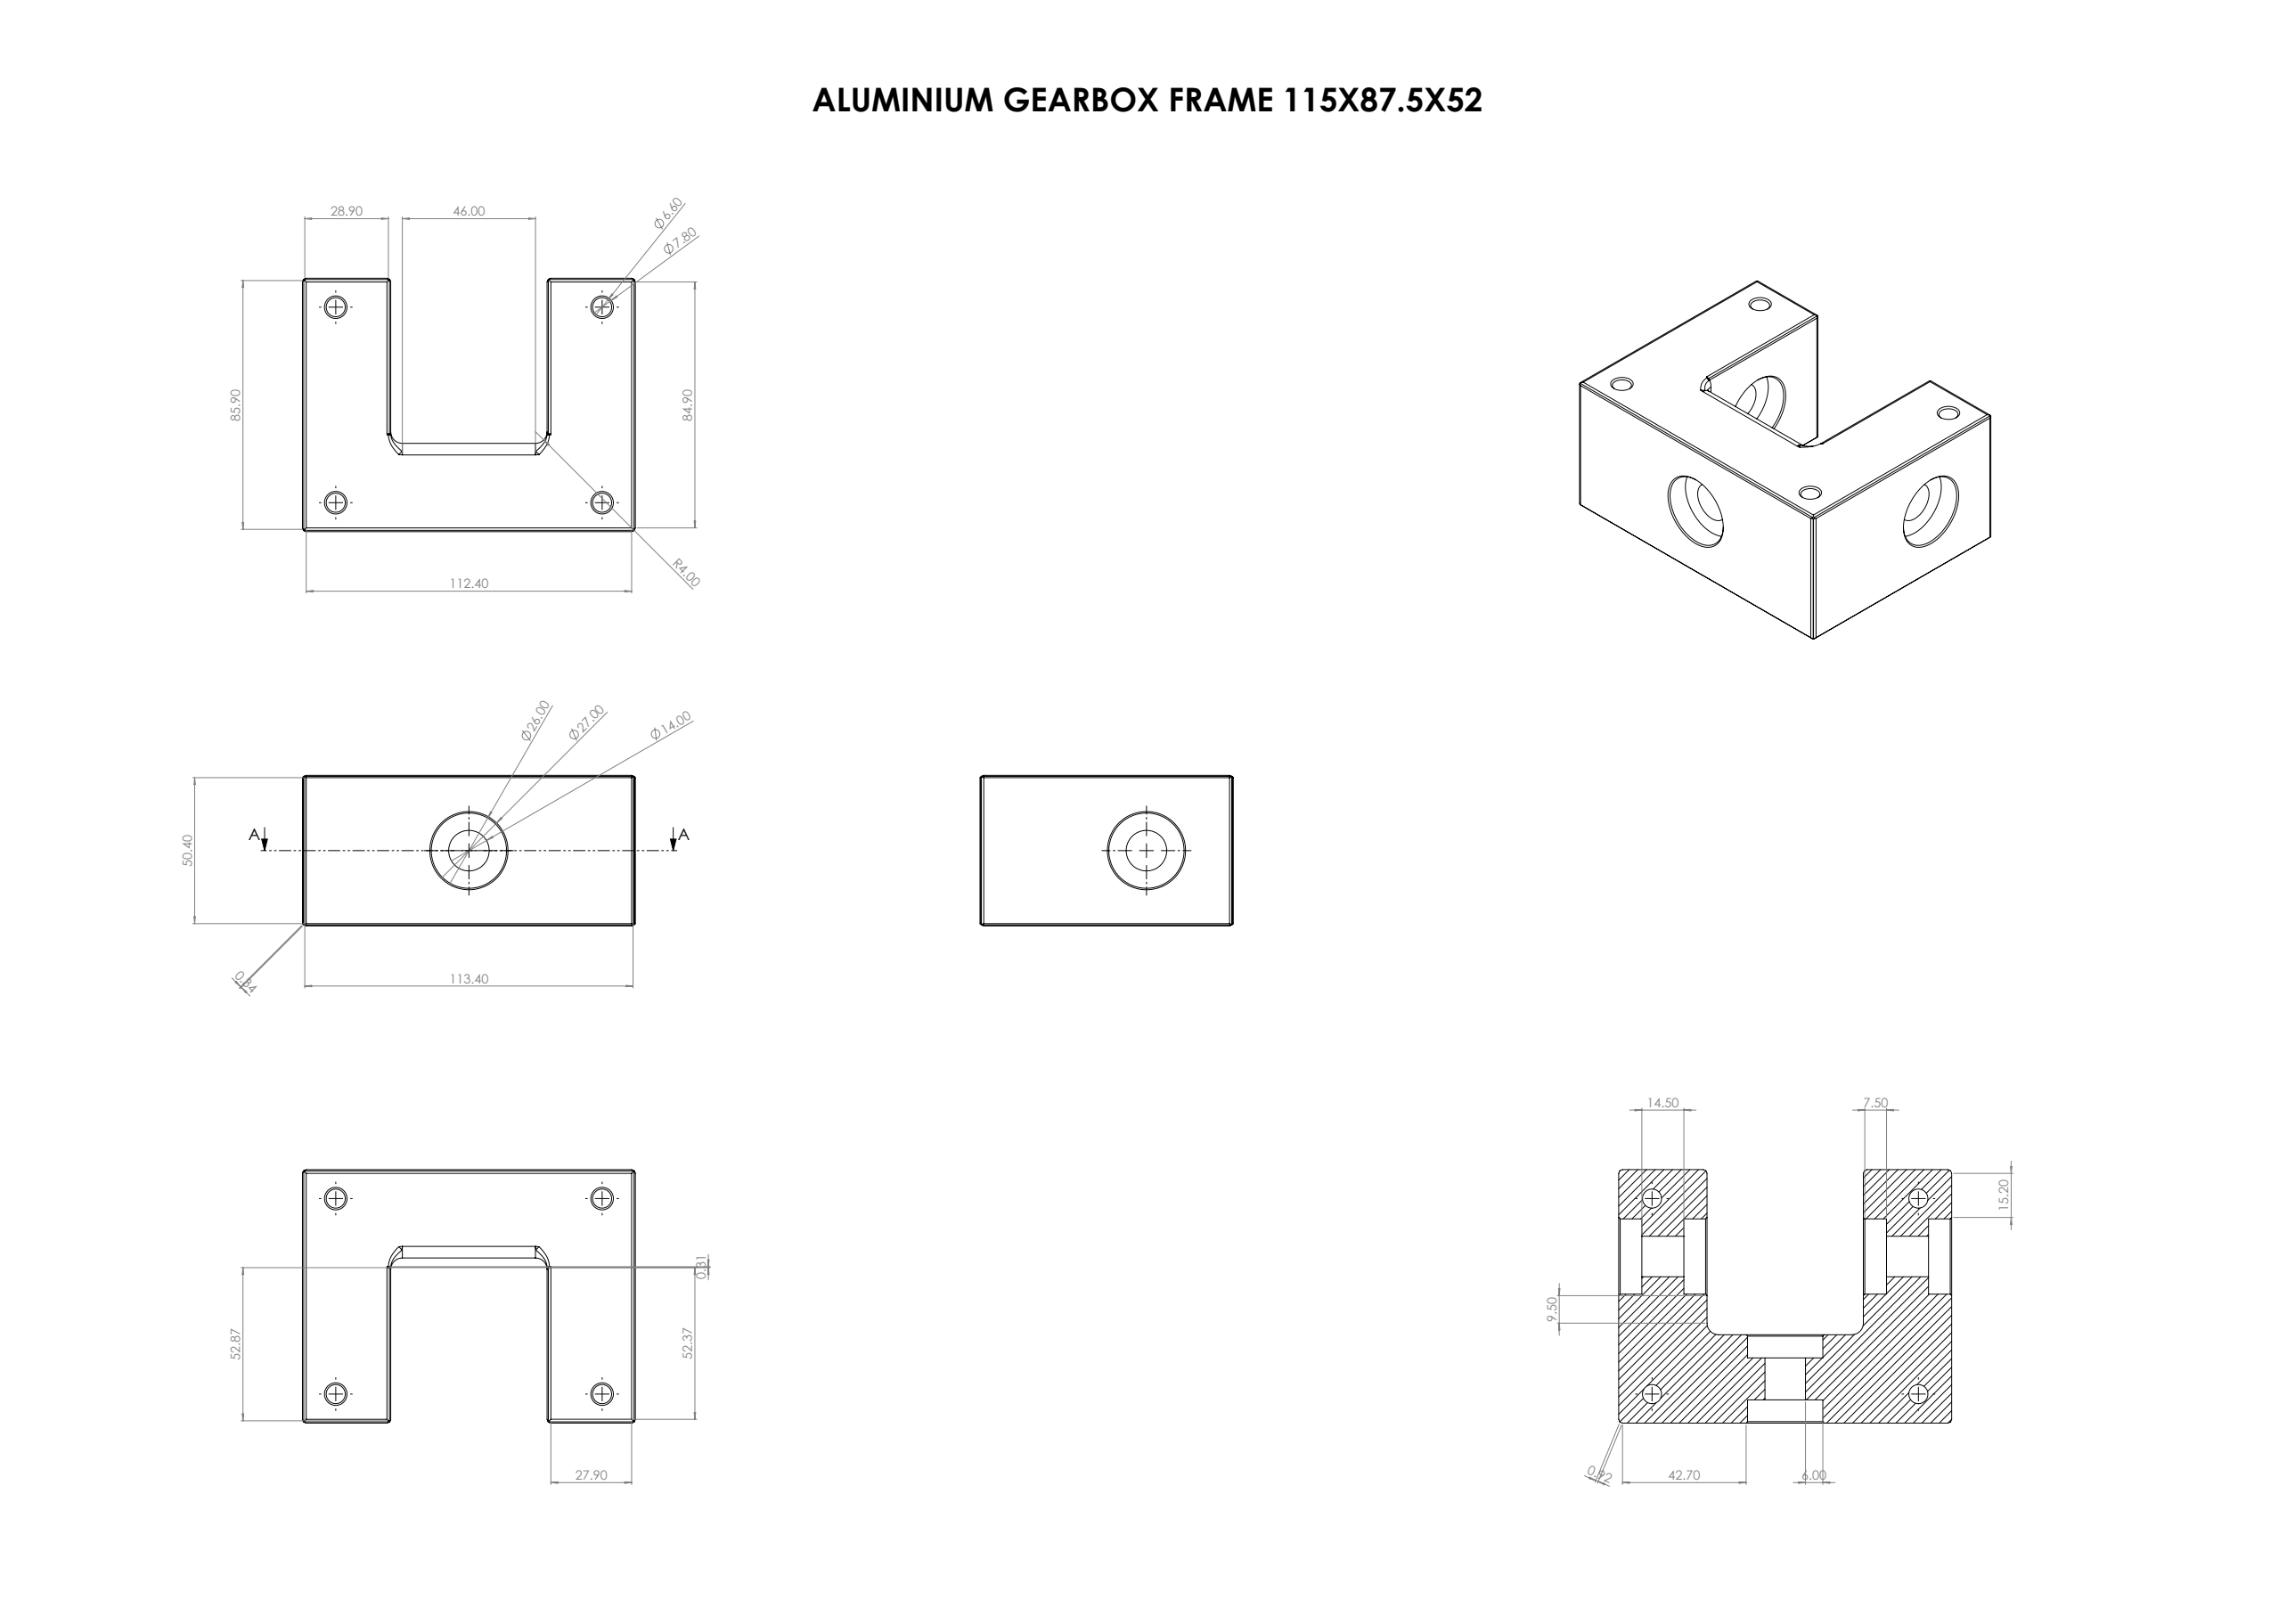
ISO-10303-21;
HEADER;
/* Generated by software containing ST-Developer
 * from STEP Tools, Inc. (www.steptools.com) 
 */

FILE_DESCRIPTION(
/* description */ (''),
/* implementation_level */ '2;1');

FILE_NAME(
/* name */ 
'01_Aluminium_Gearbox_Frame_115x87.5x52.step',
/* time_stamp */ '2026-10-22T00:21:42-07:00',
/* author */ (''),
/* organization */ (''),
/* preprocessor_version */ 'ST-DEVELOPER v20.2',
/* originating_system */ 'Autodesk Translation Framework v15.15.0.0',
/* authorisation */ '');

FILE_SCHEMA (('AUTOMOTIVE_DESIGN { 1 0 10303 214 3 1 1 }'));
ENDSEC;

DATA;
#10=MECHANICAL_DESIGN_GEOMETRIC_PRESENTATION_REPRESENTATION('',(#205),#31638);
#183=SHAPE_REPRESENTATION_RELATIONSHIP('SRR','None',#31705,#194);
#194=ADVANCED_BREP_SHAPE_REPRESENTATION('',(#216),#31627);
#205=STYLED_ITEM('',(#31809),#216);
#216=MANIFOLD_SOLID_BREP('Frame',#12480);
#227=TOROIDAL_SURFACE('',#12758,0.8,0.4);
#228=TOROIDAL_SURFACE('',#12761,0.8,0.4);
#229=TOROIDAL_SURFACE('',#12765,0.8,0.4);
#230=TOROIDAL_SURFACE('',#12770,0.8,0.4);
#246=CYLINDRICAL_SURFACE('',#12692,0.33);
#247=CYLINDRICAL_SURFACE('',#12697,0.33);
#248=CYLINDRICAL_SURFACE('',#12702,0.33);
#249=CYLINDRICAL_SURFACE('',#12707,0.33);
#250=CYLINDRICAL_SURFACE('',#12713,1.3);
#251=CYLINDRICAL_SURFACE('',#12717,0.7);
#252=CYLINDRICAL_SURFACE('',#12721,1.3);
#253=CYLINDRICAL_SURFACE('',#12727,1.3);
#254=CYLINDRICAL_SURFACE('',#12731,0.7);
#255=CYLINDRICAL_SURFACE('',#12735,1.3);
#256=CYLINDRICAL_SURFACE('',#12740,1.3);
#257=CYLINDRICAL_SURFACE('',#12744,0.7);
#258=CYLINDRICAL_SURFACE('',#12748,1.3);
#259=CYLINDRICAL_SURFACE('',#12768,0.4);
#260=CYLINDRICAL_SURFACE('',#12772,0.4);
#261=CYLINDRICAL_SURFACE('',#12773,0.4);
#262=CYLINDRICAL_SURFACE('',#12775,0.4);
#362=CONICAL_SURFACE('',#12690,0.36,0.785398163397444);
#363=CONICAL_SURFACE('',#12694,0.36,0.785398163397444);
#364=CONICAL_SURFACE('',#12695,0.36,0.785398163397444);
#365=CONICAL_SURFACE('',#12699,0.36,0.785398163397444);
#366=CONICAL_SURFACE('',#12700,0.36,0.785398163397444);
#367=CONICAL_SURFACE('',#12704,0.36,0.785398163397444);
#368=CONICAL_SURFACE('',#12705,0.36,0.785398163397444);
#369=CONICAL_SURFACE('',#12709,0.36,0.785398163397444);
#370=CONICAL_SURFACE('',#12710,1.35,0.78539816339745);
#371=CONICAL_SURFACE('',#12723,1.35,0.785398163397441);
#372=CONICAL_SURFACE('',#12725,1.35,0.785398163397451);
#373=CONICAL_SURFACE('',#12737,1.35,0.785398163397453);
#374=CONICAL_SURFACE('',#12738,1.35,0.785398163397453);
#375=CONICAL_SURFACE('',#12750,1.35,0.785398163397451);
#457=B_SPLINE_CURVE_WITH_KNOTS('',3,(#16701,#16702,#16703,#16704),
 .UNSPECIFIED.,.F.,.F.,(4,4),(0.,1.),.UNSPECIFIED.);
#458=B_SPLINE_CURVE_WITH_KNOTS('',3,(#16705,#16706,#16707,#16708),
 .UNSPECIFIED.,.F.,.F.,(4,4),(-5.39792313687514,-5.36678788880707),
 .UNSPECIFIED.);
#459=B_SPLINE_CURVE_WITH_KNOTS('',3,(#16709,#16710,#16711,#16712),
 .UNSPECIFIED.,.F.,.F.,(4,4),(5.36678788880707,5.39792313687514),
 .UNSPECIFIED.);
#460=B_SPLINE_CURVE_WITH_KNOTS('',3,(#16730,#16731,#16732,#16733),
 .UNSPECIFIED.,.F.,.F.,(4,4),(0.,1.),.UNSPECIFIED.);
#461=B_SPLINE_CURVE_WITH_KNOTS('',3,(#16734,#16735,#16736,#16737),
 .UNSPECIFIED.,.F.,.F.,(4,4),(-1.,0.),.UNSPECIFIED.);
#462=B_SPLINE_CURVE_WITH_KNOTS('',3,(#16740,#16741,#16742,#16743,#16744,
#16745,#16746,#16747,#16748),.UNSPECIFIED.,.F.,.F.,(4,1,1,1,1,1,4),(0.0919588831913347,
0.287428968788757,0.385164011587469,0.48289905438618,0.580634097184891,
0.678369139983603,0.776104182782314),.UNSPECIFIED.);
#463=B_SPLINE_CURVE_WITH_KNOTS('',3,(#16750,#16751,#16752,#16753),
 .UNSPECIFIED.,.F.,.F.,(4,4),(-1.,0.),.UNSPECIFIED.);
#464=B_SPLINE_CURVE_WITH_KNOTS('',3,(#16757,#16758,#16759,#16760),
 .UNSPECIFIED.,.F.,.F.,(4,4),(0.,1.),.UNSPECIFIED.);
#465=B_SPLINE_CURVE_WITH_KNOTS('',3,(#16762,#16763,#16764,#16765,#16766,
#16767,#16768,#16769,#16770),.UNSPECIFIED.,.F.,.F.,(4,1,1,1,2,4),(2.02212896015404,
2.13032466905734,2.23852037796064,2.34671608686394,2.56310750467053,2.7062742594363),
 .UNSPECIFIED.);
#466=B_SPLINE_CURVE_WITH_KNOTS('',3,(#16772,#16773,#16774,#16775),
 .UNSPECIFIED.,.F.,.F.,(4,4),(0.,1.),.UNSPECIFIED.);
#467=B_SPLINE_CURVE_WITH_KNOTS('',3,(#16777,#16778,#16779,#16780),
 .UNSPECIFIED.,.F.,.F.,(4,4),(-0.333212111192934,-0.302076863348255),
 .UNSPECIFIED.);
#468=B_SPLINE_CURVE_WITH_KNOTS('',3,(#16816,#16817,#16818,#16819),
 .UNSPECIFIED.,.F.,.F.,(4,4),(5.36678788880707,5.40717967697245),
 .UNSPECIFIED.);
#469=B_SPLINE_CURVE_WITH_KNOTS('',3,(#16848,#16849,#16850,#16851),
 .UNSPECIFIED.,.F.,.F.,(4,4),(-1.,0.),.UNSPECIFIED.);
#470=B_SPLINE_CURVE_WITH_KNOTS('',3,(#16852,#16853,#16854,#16855),
 .UNSPECIFIED.,.F.,.F.,(4,4),(0.302076863348255,0.333212111192934),
 .UNSPECIFIED.);
#471=B_SPLINE_CURVE_WITH_KNOTS('',3,(#16872,#16873,#16874,#16875),
 .UNSPECIFIED.,.F.,.F.,(4,4),(-1.,0.),.UNSPECIFIED.);
#472=B_SPLINE_CURVE_WITH_KNOTS('',3,(#16906,#16907,#16908,#16909),
 .UNSPECIFIED.,.F.,.F.,(4,4),(0.,1.),.UNSPECIFIED.);
#473=B_SPLINE_CURVE_WITH_KNOTS('',3,(#16910,#16911,#16912,#16913),
 .UNSPECIFIED.,.F.,.F.,(4,4),(0.302076863124856,0.333212111192934),
 .UNSPECIFIED.);
#474=B_SPLINE_CURVE_WITH_KNOTS('',3,(#16914,#16915,#16916,#16917),
 .UNSPECIFIED.,.F.,.F.,(4,4),(-0.333212111192934,-0.302076863124856),
 .UNSPECIFIED.);
#475=B_SPLINE_CURVE_WITH_KNOTS('',3,(#16935,#16936,#16937,#16938),
 .UNSPECIFIED.,.F.,.F.,(4,4),(0.,1.),.UNSPECIFIED.);
#476=B_SPLINE_CURVE_WITH_KNOTS('',3,(#16939,#16940,#16941,#16942),
 .UNSPECIFIED.,.F.,.F.,(4,4),(-1.,0.),.UNSPECIFIED.);
#477=B_SPLINE_CURVE_WITH_KNOTS('',3,(#16945,#16946,#16947,#16948,#16949,
#16950,#16951,#16952),.UNSPECIFIED.,.F.,.F.,(4,1,1,1,1,4),(0.091958883192206,
0.287428968789379,0.482899054386553,0.531766575785846,0.678369139983726,
0.776104182782313),.UNSPECIFIED.);
#478=B_SPLINE_CURVE_WITH_KNOTS('',3,(#16954,#16955,#16956,#16957),
 .UNSPECIFIED.,.F.,.F.,(4,4),(-1.,0.),.UNSPECIFIED.);
#479=B_SPLINE_CURVE_WITH_KNOTS('',3,(#16961,#16962,#16963,#16964),
 .UNSPECIFIED.,.F.,.F.,(4,4),(0.,1.),.UNSPECIFIED.);
#480=B_SPLINE_CURVE_WITH_KNOTS('',3,(#16966,#16967,#16968,#16969,#16970,
#16971,#16972,#16973,#16974),.UNSPECIFIED.,.F.,.F.,(4,1,1,1,2,4),(2.02212896015404,
2.13032466905734,2.23852037796064,2.34671608686394,2.56310750467053,2.70627425943714),
 .UNSPECIFIED.);
#481=B_SPLINE_CURVE_WITH_KNOTS('',3,(#16976,#16977,#16978,#16979),
 .UNSPECIFIED.,.F.,.F.,(4,4),(0.,1.),.UNSPECIFIED.);
#482=B_SPLINE_CURVE_WITH_KNOTS('',3,(#16981,#16982,#16983,#16984),
 .UNSPECIFIED.,.F.,.F.,(4,4),(5.36678788880707,5.39792313665175),
 .UNSPECIFIED.);
#483=B_SPLINE_CURVE_WITH_KNOTS('',3,(#17020,#17021,#17022,#17023),
 .UNSPECIFIED.,.F.,.F.,(4,4),(-0.333212111192934,-0.292820323027551),
 .UNSPECIFIED.);
#484=B_SPLINE_CURVE_WITH_KNOTS('',3,(#17057,#17058,#17059,#17060),
 .UNSPECIFIED.,.F.,.F.,(4,4),(-1.,0.),.UNSPECIFIED.);
#485=B_SPLINE_CURVE_WITH_KNOTS('',3,(#17061,#17062,#17063,#17064),
 .UNSPECIFIED.,.F.,.F.,(4,4),(-5.39792313665175,-5.36678788880707),
 .UNSPECIFIED.);
#486=B_SPLINE_CURVE_WITH_KNOTS('',3,(#17081,#17082,#17083,#17084),
 .UNSPECIFIED.,.F.,.F.,(4,4),(-1.,0.),.UNSPECIFIED.);
#487=B_SPLINE_CURVE_WITH_KNOTS('',3,(#17238,#17239,#17240,#17241),
 .UNSPECIFIED.,.F.,.F.,(4,4),(0.,1.),.UNSPECIFIED.);
#488=B_SPLINE_CURVE_WITH_KNOTS('',3,(#17242,#17243,#17244,#17245,#17246,
#17247,#17248,#17249,#17250),.UNSPECIFIED.,.F.,.F.,(4,1,1,1,1,1,4),(-0.776104182782314,
-0.678369139983603,-0.580634097184891,-0.48289905438618,-0.385164011587469,
-0.287428968788757,-0.0919588831913347),.UNSPECIFIED.);
#489=B_SPLINE_CURVE_WITH_KNOTS('',3,(#17284,#17285,#17286,#17287),
 .UNSPECIFIED.,.F.,.F.,(4,4),(0.,1.),.UNSPECIFIED.);
#490=B_SPLINE_CURVE_WITH_KNOTS('',3,(#17288,#17289,#17290,#17291,#17292,
#17293,#17294,#17295),.UNSPECIFIED.,.F.,.F.,(4,1,1,1,1,4),(-0.776104182782313,
-0.678369139983726,-0.531766575785846,-0.482899054386553,-0.287428968789379,
-0.091958883192206),.UNSPECIFIED.);
#491=B_SPLINE_CURVE_WITH_KNOTS('',3,(#17340,#17341,#17342,#17343),
 .UNSPECIFIED.,.F.,.F.,(4,4),(-1.,0.),.UNSPECIFIED.);
#492=B_SPLINE_CURVE_WITH_KNOTS('',3,(#17345,#17346,#17347,#17348,#17349,
#17350,#17351,#17352,#17353),.UNSPECIFIED.,.F.,.F.,(4,2,1,1,1,4),(-2.7062742594363,
-2.56310750467053,-2.34671608686394,-2.23852037796064,-2.13032466905734,
-2.02212896015404),.UNSPECIFIED.);
#493=B_SPLINE_CURVE_WITH_KNOTS('',3,(#17371,#17372,#17373,#17374),
 .UNSPECIFIED.,.F.,.F.,(4,4),(0.292820323027551,0.333212111192934),
 .UNSPECIFIED.);
#494=B_SPLINE_CURVE_WITH_KNOTS('',3,(#17412,#17413,#17414,#17415),
 .UNSPECIFIED.,.F.,.F.,(4,4),(-1.,0.),.UNSPECIFIED.);
#495=B_SPLINE_CURVE_WITH_KNOTS('',3,(#17417,#17418,#17419,#17420,#17421,
#17422,#17423,#17424,#17425),.UNSPECIFIED.,.F.,.F.,(4,2,1,1,1,4),(-2.70627425943714,
-2.56310750467053,-2.34671608686394,-2.23852037796064,-2.13032466905734,
-2.02212896015404),.UNSPECIFIED.);
#496=B_SPLINE_CURVE_WITH_KNOTS('',3,(#17443,#17444,#17445,#17446),
 .UNSPECIFIED.,.F.,.F.,(4,4),(-5.40717967697245,-5.36678788880707),
 .UNSPECIFIED.);
#497=B_SPLINE_CURVE_WITH_KNOTS('',3,(#17463,#17464,#17465,#17466),
 .UNSPECIFIED.,.F.,.F.,(4,4),(0.,1.),.UNSPECIFIED.);
#498=B_SPLINE_CURVE_WITH_KNOTS('',3,(#17483,#17484,#17485,#17486),
 .UNSPECIFIED.,.F.,.F.,(4,4),(0.,1.),.UNSPECIFIED.);
#499=B_SPLINE_CURVE_WITH_KNOTS('',3,(#17503,#17504,#17505,#17506),
 .UNSPECIFIED.,.F.,.F.,(4,4),(-1.,0.),.UNSPECIFIED.);
#500=B_SPLINE_CURVE_WITH_KNOTS('',3,(#17523,#17524,#17525,#17526),
 .UNSPECIFIED.,.F.,.F.,(4,4),(-1.,0.),.UNSPECIFIED.);
#1186=B_SPLINE_SURFACE_WITH_KNOTS('',3,3,((#16683,#16684,#16685,#16686),
(#16687,#16688,#16689,#16690),(#16691,#16692,#16693,#16694),(#16695,#16696,
#16697,#16698)),.UNSPECIFIED.,.F.,.F.,.F.,(4,4),(4,4),(0.,1.),(-5.39792313687514,
-5.36678788880707),.UNSPECIFIED.);
#1187=B_SPLINE_SURFACE_WITH_KNOTS('',3,3,((#16713,#16714,#16715,#16716),
(#16717,#16718,#16719,#16720),(#16721,#16722,#16723,#16724),(#16725,#16726,
#16727,#16728)),.UNSPECIFIED.,.F.,.F.,.F.,(4,4),(4,4),(0.,1.),(0.,1.),
 .UNSPECIFIED.);
#1188=B_SPLINE_SURFACE_WITH_KNOTS('',3,3,((#16798,#16799,#16800,#16801),
(#16802,#16803,#16804,#16805),(#16806,#16807,#16808,#16809),(#16810,#16811,
#16812,#16813)),.UNSPECIFIED.,.F.,.F.,.F.,(4,4),(4,4),(0.,1.),(-5.40717967697245,
-5.36678788880707),.UNSPECIFIED.);
#1189=B_SPLINE_SURFACE_WITH_KNOTS('',3,3,((#16831,#16832,#16833,#16834),
(#16835,#16836,#16837,#16838),(#16839,#16840,#16841,#16842),(#16843,#16844,
#16845,#16846)),.UNSPECIFIED.,.F.,.F.,.F.,(4,4),(4,4),(0.,1.),(-0.333212111192934,
-0.302076863348255),.UNSPECIFIED.);
#1190=B_SPLINE_SURFACE_WITH_KNOTS('',3,3,((#16856,#16857,#16858,#16859),
(#16860,#16861,#16862,#16863),(#16864,#16865,#16866,#16867),(#16868,#16869,
#16870,#16871)),.UNSPECIFIED.,.F.,.F.,.F.,(4,4),(4,4),(0.,1.),(0.,1.),
 .UNSPECIFIED.);
#1191=B_SPLINE_SURFACE_WITH_KNOTS('',3,3,((#16888,#16889,#16890,#16891),
(#16892,#16893,#16894,#16895),(#16896,#16897,#16898,#16899),(#16900,#16901,
#16902,#16903)),.UNSPECIFIED.,.F.,.F.,.F.,(4,4),(4,4),(0.,1.),(0.302076863124856,
0.333212111192934),.UNSPECIFIED.);
#1192=B_SPLINE_SURFACE_WITH_KNOTS('',3,3,((#16918,#16919,#16920,#16921),
(#16922,#16923,#16924,#16925),(#16926,#16927,#16928,#16929),(#16930,#16931,
#16932,#16933)),.UNSPECIFIED.,.F.,.F.,.F.,(4,4),(4,4),(0.,1.),(0.,1.),
 .UNSPECIFIED.);
#1193=B_SPLINE_SURFACE_WITH_KNOTS('',3,3,((#17002,#17003,#17004,#17005),
(#17006,#17007,#17008,#17009),(#17010,#17011,#17012,#17013),(#17014,#17015,
#17016,#17017)),.UNSPECIFIED.,.F.,.F.,.F.,(4,4),(4,4),(0.,1.),(0.292820323027551,
0.333212111192934),.UNSPECIFIED.);
#1194=B_SPLINE_SURFACE_WITH_KNOTS('',3,3,((#17040,#17041,#17042,#17043),
(#17044,#17045,#17046,#17047),(#17048,#17049,#17050,#17051),(#17052,#17053,
#17054,#17055)),.UNSPECIFIED.,.F.,.F.,.F.,(4,4),(4,4),(0.,1.),(5.36678788880707,
5.39792313665175),.UNSPECIFIED.);
#1195=B_SPLINE_SURFACE_WITH_KNOTS('',3,3,((#17065,#17066,#17067,#17068),
(#17069,#17070,#17071,#17072),(#17073,#17074,#17075,#17076),(#17077,#17078,
#17079,#17080)),.UNSPECIFIED.,.F.,.F.,.F.,(4,4),(4,4),(0.,1.),(0.,1.),
 .UNSPECIFIED.);
#1196=B_SPLINE_SURFACE_WITH_KNOTS('',3,3,((#17201,#17202,#17203,#17204,
#17205,#17206,#17207,#17208,#17209),(#17210,#17211,#17212,#17213,#17214,
#17215,#17216,#17217,#17218),(#17219,#17220,#17221,#17222,#17223,#17224,
#17225,#17226,#17227),(#17228,#17229,#17230,#17231,#17232,#17233,#17234,
#17235,#17236)),.UNSPECIFIED.,.F.,.F.,.F.,(4,4),(4,1,1,1,1,1,4),(0.,1.),
(0.0919588831913347,0.287428968788757,0.385164011587469,0.48289905438618,
0.580634097184891,0.678369139983603,0.776104182782314),.UNSPECIFIED.);
#1197=B_SPLINE_SURFACE_WITH_KNOTS('',3,3,((#17251,#17252,#17253,#17254,
#17255,#17256,#17257,#17258),(#17259,#17260,#17261,#17262,#17263,#17264,
#17265,#17266),(#17267,#17268,#17269,#17270,#17271,#17272,#17273,#17274),
(#17275,#17276,#17277,#17278,#17279,#17280,#17281,#17282)),
 .UNSPECIFIED.,.F.,.F.,.F.,(4,4),(4,1,1,1,1,4),(0.,1.),(0.091958883192206,
0.287428968789379,0.482899054386553,0.531766575785846,0.678369139983726,
0.776104182782313),.UNSPECIFIED.);
#1198=B_SPLINE_SURFACE_WITH_KNOTS('',3,3,((#17303,#17304,#17305,#17306,
#17307,#17308,#17309,#17310,#17311),(#17312,#17313,#17314,#17315,#17316,
#17317,#17318,#17319,#17320),(#17321,#17322,#17323,#17324,#17325,#17326,
#17327,#17328,#17329),(#17330,#17331,#17332,#17333,#17334,#17335,#17336,
#17337,#17338)),.UNSPECIFIED.,.F.,.F.,.F.,(4,4),(4,1,1,1,2,4),(0.,1.),(2.02212896015404,
2.13032466905734,2.23852037796064,2.34671608686394,2.56310750467053,2.7062742594363),
 .UNSPECIFIED.);
#1199=B_SPLINE_SURFACE_WITH_KNOTS('',3,3,((#17355,#17356,#17357,#17358),
(#17359,#17360,#17361,#17362),(#17363,#17364,#17365,#17366),(#17367,#17368,
#17369,#17370)),.UNSPECIFIED.,.F.,.F.,.F.,(4,4),(4,4),(0.,1.),(-0.333212111192934,
-0.292820323027551),.UNSPECIFIED.);
#1200=B_SPLINE_SURFACE_WITH_KNOTS('',3,3,((#17375,#17376,#17377,#17378,
#17379,#17380,#17381,#17382,#17383),(#17384,#17385,#17386,#17387,#17388,
#17389,#17390,#17391,#17392),(#17393,#17394,#17395,#17396,#17397,#17398,
#17399,#17400,#17401),(#17402,#17403,#17404,#17405,#17406,#17407,#17408,
#17409,#17410)),.UNSPECIFIED.,.F.,.F.,.F.,(4,4),(4,1,1,1,2,4),(0.,1.),(2.02212896015404,
2.13032466905734,2.23852037796064,2.34671608686394,2.56310750467053,2.70627425943714),
 .UNSPECIFIED.);
#1201=B_SPLINE_SURFACE_WITH_KNOTS('',3,3,((#17427,#17428,#17429,#17430),
(#17431,#17432,#17433,#17434),(#17435,#17436,#17437,#17438),(#17439,#17440,
#17441,#17442)),.UNSPECIFIED.,.F.,.F.,.F.,(4,4),(4,4),(0.,1.),(5.36678788880707,
5.40717967697245),.UNSPECIFIED.);
#1202=B_SPLINE_SURFACE_WITH_KNOTS('',3,3,((#17447,#17448,#17449,#17450),
(#17451,#17452,#17453,#17454),(#17455,#17456,#17457,#17458),(#17459,#17460,
#17461,#17462)),.UNSPECIFIED.,.F.,.F.,.F.,(4,4),(4,4),(0.,1.),(0.,1.),
 .UNSPECIFIED.);
#1203=B_SPLINE_SURFACE_WITH_KNOTS('',3,3,((#17467,#17468,#17469,#17470),
(#17471,#17472,#17473,#17474),(#17475,#17476,#17477,#17478),(#17479,#17480,
#17481,#17482)),.UNSPECIFIED.,.F.,.F.,.F.,(4,4),(4,4),(0.,1.),(0.,1.),
 .UNSPECIFIED.);
#1204=B_SPLINE_SURFACE_WITH_KNOTS('',3,3,((#17487,#17488,#17489,#17490),
(#17491,#17492,#17493,#17494),(#17495,#17496,#17497,#17498),(#17499,#17500,
#17501,#17502)),.UNSPECIFIED.,.F.,.F.,.F.,(4,4),(4,4),(0.,1.),(0.,1.),
 .UNSPECIFIED.);
#1205=B_SPLINE_SURFACE_WITH_KNOTS('',3,3,((#17507,#17508,#17509,#17510),
(#17511,#17512,#17513,#17514),(#17515,#17516,#17517,#17518),(#17519,#17520,
#17521,#17522)),.UNSPECIFIED.,.F.,.F.,.F.,(4,4),(4,4),(0.,1.),(0.,1.),
 .UNSPECIFIED.);
#1340=FACE_BOUND('',#2515,.T.);
#1341=FACE_BOUND('',#2527,.T.);
#1342=FACE_BOUND('',#2540,.T.);
#1343=FACE_BOUND('',#2556,.T.);
#1344=FACE_BOUND('',#2564,.T.);
#1345=FACE_BOUND('',#2565,.T.);
#1346=FACE_BOUND('',#2566,.T.);
#1347=FACE_BOUND('',#2567,.T.);
#1348=FACE_BOUND('',#2581,.T.);
#1349=FACE_BOUND('',#2582,.T.);
#1350=FACE_BOUND('',#2583,.T.);
#1351=FACE_BOUND('',#2584,.T.);
#1352=FACE_BOUND('',#2609,.T.);
#1353=FACE_BOUND('',#2612,.T.);
#1354=FACE_BOUND('',#2618,.T.);
#1355=FACE_BOUND('',#2621,.T.);
#1356=FACE_BOUND('',#2627,.T.);
#1357=FACE_BOUND('',#2630,.T.);
#1358=FACE_BOUND('',#2653,.T.);
#1359=FACE_BOUND('',#2660,.T.);
#1405=CIRCLE('',#12617,0.8);
#1406=CIRCLE('',#12618,0.8);
#1407=CIRCLE('',#12619,1.35);
#1408=CIRCLE('',#12631,1.35);
#1409=CIRCLE('',#12644,1.35);
#1410=CIRCLE('',#12660,0.8);
#1411=CIRCLE('',#12661,0.8);
#1412=CIRCLE('',#12662,1.35);
#1413=CIRCLE('',#12668,0.39);
#1414=CIRCLE('',#12669,0.39);
#1415=CIRCLE('',#12670,0.39);
#1416=CIRCLE('',#12671,0.39);
#1417=CIRCLE('',#12680,0.39);
#1418=CIRCLE('',#12681,0.39);
#1419=CIRCLE('',#12682,0.39);
#1420=CIRCLE('',#12683,0.39);
#1421=CIRCLE('',#12691,0.33);
#1422=CIRCLE('',#12693,0.33);
#1423=CIRCLE('',#12696,0.33);
#1424=CIRCLE('',#12698,0.33);
#1425=CIRCLE('',#12701,0.33);
#1426=CIRCLE('',#12703,0.33);
#1427=CIRCLE('',#12706,0.33);
#1428=CIRCLE('',#12708,0.33);
#1429=CIRCLE('',#12711,1.35);
#1430=CIRCLE('',#12712,1.3);
#1431=CIRCLE('',#12714,1.3);
#1432=CIRCLE('',#12716,0.7);
#1433=CIRCLE('',#12718,0.7);
#1434=CIRCLE('',#12720,1.3);
#1435=CIRCLE('',#12722,1.3);
#1436=CIRCLE('',#12724,1.35);
#1437=CIRCLE('',#12726,1.3);
#1438=CIRCLE('',#12728,1.3);
#1439=CIRCLE('',#12730,0.7);
#1440=CIRCLE('',#12732,0.7);
#1441=CIRCLE('',#12734,1.3);
#1442=CIRCLE('',#12736,1.3);
#1443=CIRCLE('',#12739,1.3);
#1444=CIRCLE('',#12741,1.3);
#1445=CIRCLE('',#12743,0.7);
#1446=CIRCLE('',#12745,0.7);
#1447=CIRCLE('',#12747,1.3);
#1448=CIRCLE('',#12749,1.3);
#1449=CIRCLE('',#12759,0.4);
#1450=CIRCLE('',#12760,0.4);
#1451=CIRCLE('',#12762,0.4);
#1452=CIRCLE('',#12763,0.4);
#1453=CIRCLE('',#12766,0.4);
#1454=CIRCLE('',#12767,0.4);
#1455=CIRCLE('',#12769,0.4);
#1456=CIRCLE('',#12771,0.4);
#1819=FACE_OUTER_BOUND('',#2513,.T.);
#1820=FACE_OUTER_BOUND('',#2514,.T.);
#1821=FACE_OUTER_BOUND('',#2516,.T.);
#1822=FACE_OUTER_BOUND('',#2517,.T.);
#1823=FACE_OUTER_BOUND('',#2518,.T.);
#1824=FACE_OUTER_BOUND('',#2519,.T.);
#1825=FACE_OUTER_BOUND('',#2520,.T.);
#1826=FACE_OUTER_BOUND('',#2521,.T.);
#1827=FACE_OUTER_BOUND('',#2522,.T.);
#1828=FACE_OUTER_BOUND('',#2523,.T.);
#1829=FACE_OUTER_BOUND('',#2524,.T.);
#1830=FACE_OUTER_BOUND('',#2525,.T.);
#1831=FACE_OUTER_BOUND('',#2526,.T.);
#1832=FACE_OUTER_BOUND('',#2528,.T.);
#1833=FACE_OUTER_BOUND('',#2529,.T.);
#1834=FACE_OUTER_BOUND('',#2530,.T.);
#1835=FACE_OUTER_BOUND('',#2531,.T.);
#1836=FACE_OUTER_BOUND('',#2532,.T.);
#1837=FACE_OUTER_BOUND('',#2533,.T.);
#1838=FACE_OUTER_BOUND('',#2534,.T.);
#1839=FACE_OUTER_BOUND('',#2535,.T.);
#1840=FACE_OUTER_BOUND('',#2536,.T.);
#1841=FACE_OUTER_BOUND('',#2537,.T.);
#1842=FACE_OUTER_BOUND('',#2538,.T.);
#1843=FACE_OUTER_BOUND('',#2539,.T.);
#1844=FACE_OUTER_BOUND('',#2541,.T.);
#1845=FACE_OUTER_BOUND('',#2542,.T.);
#1846=FACE_OUTER_BOUND('',#2543,.T.);
#1847=FACE_OUTER_BOUND('',#2544,.T.);
#1848=FACE_OUTER_BOUND('',#2545,.T.);
#1849=FACE_OUTER_BOUND('',#2546,.T.);
#1850=FACE_OUTER_BOUND('',#2547,.T.);
#1851=FACE_OUTER_BOUND('',#2548,.T.);
#1852=FACE_OUTER_BOUND('',#2549,.T.);
#1853=FACE_OUTER_BOUND('',#2550,.T.);
#1854=FACE_OUTER_BOUND('',#2551,.T.);
#1855=FACE_OUTER_BOUND('',#2552,.T.);
#1856=FACE_OUTER_BOUND('',#2553,.T.);
#1857=FACE_OUTER_BOUND('',#2554,.T.);
#1858=FACE_OUTER_BOUND('',#2555,.T.);
#1859=FACE_OUTER_BOUND('',#2557,.T.);
#1860=FACE_OUTER_BOUND('',#2558,.T.);
#1861=FACE_OUTER_BOUND('',#2559,.T.);
#1862=FACE_OUTER_BOUND('',#2560,.T.);
#1863=FACE_OUTER_BOUND('',#2561,.T.);
#1864=FACE_OUTER_BOUND('',#2562,.T.);
#1865=FACE_OUTER_BOUND('',#2563,.T.);
#1866=FACE_OUTER_BOUND('',#2568,.T.);
#1867=FACE_OUTER_BOUND('',#2569,.T.);
#1868=FACE_OUTER_BOUND('',#2570,.T.);
#1869=FACE_OUTER_BOUND('',#2571,.T.);
#1870=FACE_OUTER_BOUND('',#2572,.T.);
#1871=FACE_OUTER_BOUND('',#2573,.T.);
#1872=FACE_OUTER_BOUND('',#2574,.T.);
#1873=FACE_OUTER_BOUND('',#2575,.T.);
#1874=FACE_OUTER_BOUND('',#2576,.T.);
#1875=FACE_OUTER_BOUND('',#2577,.T.);
#1876=FACE_OUTER_BOUND('',#2578,.T.);
#1877=FACE_OUTER_BOUND('',#2579,.T.);
#1878=FACE_OUTER_BOUND('',#2580,.T.);
#1879=FACE_OUTER_BOUND('',#2585,.T.);
#1880=FACE_OUTER_BOUND('',#2586,.T.);
#1881=FACE_OUTER_BOUND('',#2587,.T.);
#1882=FACE_OUTER_BOUND('',#2588,.T.);
#1883=FACE_OUTER_BOUND('',#2589,.T.);
#1884=FACE_OUTER_BOUND('',#2590,.T.);
#1885=FACE_OUTER_BOUND('',#2591,.T.);
#1886=FACE_OUTER_BOUND('',#2592,.T.);
#1887=FACE_OUTER_BOUND('',#2593,.T.);
#1888=FACE_OUTER_BOUND('',#2594,.T.);
#1889=FACE_OUTER_BOUND('',#2595,.T.);
#1890=FACE_OUTER_BOUND('',#2596,.T.);
#1891=FACE_OUTER_BOUND('',#2597,.T.);
#1892=FACE_OUTER_BOUND('',#2598,.T.);
#1893=FACE_OUTER_BOUND('',#2599,.T.);
#1894=FACE_OUTER_BOUND('',#2600,.T.);
#1895=FACE_OUTER_BOUND('',#2601,.T.);
#1896=FACE_OUTER_BOUND('',#2602,.T.);
#1897=FACE_OUTER_BOUND('',#2603,.T.);
#1898=FACE_OUTER_BOUND('',#2604,.T.);
#1899=FACE_OUTER_BOUND('',#2605,.T.);
#1900=FACE_OUTER_BOUND('',#2606,.T.);
#1901=FACE_OUTER_BOUND('',#2607,.T.);
#1902=FACE_OUTER_BOUND('',#2608,.T.);
#1903=FACE_OUTER_BOUND('',#2610,.T.);
#1904=FACE_OUTER_BOUND('',#2611,.T.);
#1905=FACE_OUTER_BOUND('',#2613,.T.);
#1906=FACE_OUTER_BOUND('',#2614,.T.);
#1907=FACE_OUTER_BOUND('',#2615,.T.);
#1908=FACE_OUTER_BOUND('',#2616,.T.);
#1909=FACE_OUTER_BOUND('',#2617,.T.);
#1910=FACE_OUTER_BOUND('',#2619,.T.);
#1911=FACE_OUTER_BOUND('',#2620,.T.);
#1912=FACE_OUTER_BOUND('',#2622,.T.);
#1913=FACE_OUTER_BOUND('',#2623,.T.);
#1914=FACE_OUTER_BOUND('',#2624,.T.);
#1915=FACE_OUTER_BOUND('',#2625,.T.);
#1916=FACE_OUTER_BOUND('',#2626,.T.);
#1917=FACE_OUTER_BOUND('',#2628,.T.);
#1918=FACE_OUTER_BOUND('',#2629,.T.);
#1919=FACE_OUTER_BOUND('',#2631,.T.);
#1920=FACE_OUTER_BOUND('',#2632,.T.);
#1921=FACE_OUTER_BOUND('',#2633,.T.);
#1922=FACE_OUTER_BOUND('',#2634,.T.);
#1923=FACE_OUTER_BOUND('',#2635,.T.);
#1924=FACE_OUTER_BOUND('',#2636,.T.);
#1925=FACE_OUTER_BOUND('',#2637,.T.);
#1926=FACE_OUTER_BOUND('',#2638,.T.);
#1927=FACE_OUTER_BOUND('',#2639,.T.);
#1928=FACE_OUTER_BOUND('',#2640,.T.);
#1929=FACE_OUTER_BOUND('',#2641,.T.);
#1930=FACE_OUTER_BOUND('',#2642,.T.);
#1931=FACE_OUTER_BOUND('',#2643,.T.);
#1932=FACE_OUTER_BOUND('',#2644,.T.);
#1933=FACE_OUTER_BOUND('',#2645,.T.);
#1934=FACE_OUTER_BOUND('',#2646,.T.);
#1935=FACE_OUTER_BOUND('',#2647,.T.);
#1936=FACE_OUTER_BOUND('',#2648,.T.);
#1937=FACE_OUTER_BOUND('',#2649,.T.);
#1938=FACE_OUTER_BOUND('',#2650,.T.);
#1939=FACE_OUTER_BOUND('',#2651,.T.);
#1940=FACE_OUTER_BOUND('',#2652,.T.);
#1941=FACE_OUTER_BOUND('',#2654,.T.);
#1942=FACE_OUTER_BOUND('',#2655,.T.);
#1943=FACE_OUTER_BOUND('',#2656,.T.);
#1944=FACE_OUTER_BOUND('',#2657,.T.);
#1945=FACE_OUTER_BOUND('',#2658,.T.);
#1946=FACE_OUTER_BOUND('',#2659,.T.);
#1947=FACE_OUTER_BOUND('',#2661,.T.);
#2513=EDGE_LOOP('',(#7753,#7754,#7755,#7756,#7757,#7758));
#2514=EDGE_LOOP('',(#7759,#7760,#7761,#7762,#7763,#7764));
#2515=EDGE_LOOP('',(#7765));
#2516=EDGE_LOOP('',(#7766,#7767,#7768,#7769,#7770));
#2517=EDGE_LOOP('',(#7771,#7772,#7773,#7774,#7775,#7776,#7777));
#2518=EDGE_LOOP('',(#7778,#7779,#7780,#7781,#7782,#7783));
#2519=EDGE_LOOP('',(#7784,#7785,#7786,#7787));
#2520=EDGE_LOOP('',(#7788,#7789,#7790,#7791,#7792,#7793));
#2521=EDGE_LOOP('',(#7794,#7795,#7796,#7797,#7798,#7799,#7800));
#2522=EDGE_LOOP('',(#7801,#7802,#7803,#7804,#7805,#7806));
#2523=EDGE_LOOP('',(#7807,#7808,#7809,#7810,#7811,#7812));
#2524=EDGE_LOOP('',(#7813,#7814,#7815,#7816,#7817,#7818,#7819));
#2525=EDGE_LOOP('',(#7820,#7821,#7822,#7823,#7824,#7825));
#2526=EDGE_LOOP('',(#7826,#7827,#7828,#7829));
#2527=EDGE_LOOP('',(#7830));
#2528=EDGE_LOOP('',(#7831,#7832,#7833,#7834,#7835,#7836));
#2529=EDGE_LOOP('',(#7837,#7838,#7839,#7840,#7841,#7842,#7843));
#2530=EDGE_LOOP('',(#7844,#7845,#7846,#7847,#7848,#7849));
#2531=EDGE_LOOP('',(#7850,#7851,#7852,#7853,#7854,#7855));
#2532=EDGE_LOOP('',(#7856,#7857,#7858,#7859,#7860,#7861,#7862));
#2533=EDGE_LOOP('',(#7863,#7864,#7865,#7866));
#2534=EDGE_LOOP('',(#7867,#7868,#7869,#7870,#7871,#7872));
#2535=EDGE_LOOP('',(#7873,#7874,#7875,#7876,#7877,#7878));
#2536=EDGE_LOOP('',(#7879,#7880,#7881,#7882,#7883,#7884));
#2537=EDGE_LOOP('',(#7885,#7886,#7887,#7888,#7889,#7890,#7891));
#2538=EDGE_LOOP('',(#7892,#7893,#7894,#7895,#7896,#7897));
#2539=EDGE_LOOP('',(#7898,#7899,#7900,#7901));
#2540=EDGE_LOOP('',(#7902));
#2541=EDGE_LOOP('',(#7903,#7904,#7905,#7906,#7907,#7908));
#2542=EDGE_LOOP('',(#7909,#7910,#7911,#7912));
#2543=EDGE_LOOP('',(#7913,#7914,#7915,#7916,#7917,#7918,#7919));
#2544=EDGE_LOOP('',(#7920,#7921,#7922,#7923,#7924,#7925));
#2545=EDGE_LOOP('',(#7926,#7927,#7928,#7929,#7930,#7931));
#2546=EDGE_LOOP('',(#7932,#7933,#7934,#7935,#7936,#7937,#7938));
#2547=EDGE_LOOP('',(#7939,#7940,#7941,#7942,#7943,#7944));
#2548=EDGE_LOOP('',(#7945,#7946,#7947,#7948));
#2549=EDGE_LOOP('',(#7949,#7950,#7951,#7952,#7953,#7954));
#2550=EDGE_LOOP('',(#7955,#7956,#7957,#7958,#7959,#7960,#7961));
#2551=EDGE_LOOP('',(#7962,#7963,#7964,#7965,#7966,#7967));
#2552=EDGE_LOOP('',(#7968,#7969,#7970,#7971,#7972,#7973));
#2553=EDGE_LOOP('',(#7974,#7975,#7976,#7977,#7978,#7979,#7980));
#2554=EDGE_LOOP('',(#7981,#7982,#7983,#7984,#7985,#7986));
#2555=EDGE_LOOP('',(#7987,#7988,#7989,#7990,#7991,#7992));
#2556=EDGE_LOOP('',(#7993));
#2557=EDGE_LOOP('',(#7994,#7995,#7996,#7997,#7998));
#2558=EDGE_LOOP('',(#7999,#8000,#8001,#8002,#8003,#8004,#8005));
#2559=EDGE_LOOP('',(#8006,#8007,#8008,#8009,#8010,#8011));
#2560=EDGE_LOOP('',(#8012,#8013,#8014,#8015,#8016));
#2561=EDGE_LOOP('',(#8017,#8018,#8019,#8020));
#2562=EDGE_LOOP('',(#8021,#8022,#8023));
#2563=EDGE_LOOP('',(#8024,#8025,#8026,#8027,#8028,#8029,#8030,#8031,#8032,
#8033,#8034,#8035,#8036,#8037,#8038,#8039));
#2564=EDGE_LOOP('',(#8040));
#2565=EDGE_LOOP('',(#8041));
#2566=EDGE_LOOP('',(#8042));
#2567=EDGE_LOOP('',(#8043));
#2568=EDGE_LOOP('',(#8044,#8045,#8046,#8047,#8048));
#2569=EDGE_LOOP('',(#8049,#8050,#8051,#8052,#8053,#8054));
#2570=EDGE_LOOP('',(#8055,#8056,#8057,#8058,#8059,#8060));
#2571=EDGE_LOOP('',(#8061,#8062,#8063,#8064,#8065,#8066));
#2572=EDGE_LOOP('',(#8067,#8068,#8069,#8070,#8071,#8072));
#2573=EDGE_LOOP('',(#8073,#8074,#8075,#8076,#8077));
#2574=EDGE_LOOP('',(#8078,#8079,#8080,#8081));
#2575=EDGE_LOOP('',(#8082,#8083,#8084));
#2576=EDGE_LOOP('',(#8085,#8086,#8087,#8088,#8089,#8090));
#2577=EDGE_LOOP('',(#8091,#8092,#8093,#8094,#8095));
#2578=EDGE_LOOP('',(#8096,#8097,#8098,#8099));
#2579=EDGE_LOOP('',(#8100,#8101,#8102));
#2580=EDGE_LOOP('',(#8103,#8104,#8105,#8106,#8107,#8108,#8109,#8110,#8111,
#8112,#8113,#8114,#8115,#8116,#8117,#8118));
#2581=EDGE_LOOP('',(#8119));
#2582=EDGE_LOOP('',(#8120));
#2583=EDGE_LOOP('',(#8121));
#2584=EDGE_LOOP('',(#8122));
#2585=EDGE_LOOP('',(#8123,#8124,#8125,#8126,#8127));
#2586=EDGE_LOOP('',(#8128,#8129,#8130,#8131,#8132,#8133));
#2587=EDGE_LOOP('',(#8134,#8135,#8136,#8137,#8138,#8139));
#2588=EDGE_LOOP('',(#8140,#8141,#8142,#8143,#8144,#8145,#8146));
#2589=EDGE_LOOP('',(#8147,#8148,#8149,#8150,#8151,#8152));
#2590=EDGE_LOOP('',(#8153,#8154,#8155,#8156,#8157,#8158));
#2591=EDGE_LOOP('',(#8159,#8160,#8161,#8162,#8163));
#2592=EDGE_LOOP('',(#8164,#8165,#8166,#8167));
#2593=EDGE_LOOP('',(#8168,#8169,#8170));
#2594=EDGE_LOOP('',(#8171,#8172,#8173,#8174));
#2595=EDGE_LOOP('',(#8175,#8176,#8177,#8178));
#2596=EDGE_LOOP('',(#8179,#8180,#8181,#8182));
#2597=EDGE_LOOP('',(#8183,#8184,#8185,#8186));
#2598=EDGE_LOOP('',(#8187,#8188,#8189,#8190));
#2599=EDGE_LOOP('',(#8191,#8192,#8193,#8194));
#2600=EDGE_LOOP('',(#8195,#8196,#8197,#8198));
#2601=EDGE_LOOP('',(#8199,#8200,#8201,#8202));
#2602=EDGE_LOOP('',(#8203,#8204,#8205,#8206));
#2603=EDGE_LOOP('',(#8207,#8208,#8209,#8210));
#2604=EDGE_LOOP('',(#8211,#8212,#8213,#8214));
#2605=EDGE_LOOP('',(#8215,#8216,#8217,#8218));
#2606=EDGE_LOOP('',(#8219,#8220,#8221,#8222));
#2607=EDGE_LOOP('',(#8223,#8224,#8225,#8226));
#2608=EDGE_LOOP('',(#8227));
#2609=EDGE_LOOP('',(#8228));
#2610=EDGE_LOOP('',(#8229,#8230,#8231,#8232));
#2611=EDGE_LOOP('',(#8233));
#2612=EDGE_LOOP('',(#8234));
#2613=EDGE_LOOP('',(#8235,#8236,#8237,#8238));
#2614=EDGE_LOOP('',(#8239,#8240,#8241,#8242));
#2615=EDGE_LOOP('',(#8243,#8244,#8245,#8246));
#2616=EDGE_LOOP('',(#8247,#8248,#8249,#8250));
#2617=EDGE_LOOP('',(#8251));
#2618=EDGE_LOOP('',(#8252));
#2619=EDGE_LOOP('',(#8253,#8254,#8255,#8256));
#2620=EDGE_LOOP('',(#8257));
#2621=EDGE_LOOP('',(#8258));
#2622=EDGE_LOOP('',(#8259,#8260,#8261,#8262));
#2623=EDGE_LOOP('',(#8263,#8264,#8265,#8266));
#2624=EDGE_LOOP('',(#8267,#8268,#8269,#8270));
#2625=EDGE_LOOP('',(#8271,#8272,#8273,#8274));
#2626=EDGE_LOOP('',(#8275));
#2627=EDGE_LOOP('',(#8276));
#2628=EDGE_LOOP('',(#8277,#8278,#8279,#8280));
#2629=EDGE_LOOP('',(#8281));
#2630=EDGE_LOOP('',(#8282));
#2631=EDGE_LOOP('',(#8283,#8284,#8285,#8286));
#2632=EDGE_LOOP('',(#8287,#8288,#8289,#8290));
#2633=EDGE_LOOP('',(#8291,#8292,#8293,#8294));
#2634=EDGE_LOOP('',(#8295,#8296,#8297,#8298));
#2635=EDGE_LOOP('',(#8299,#8300,#8301,#8302));
#2636=EDGE_LOOP('',(#8303,#8304,#8305,#8306));
#2637=EDGE_LOOP('',(#8307,#8308,#8309,#8310));
#2638=EDGE_LOOP('',(#8311,#8312,#8313,#8314));
#2639=EDGE_LOOP('',(#8315,#8316,#8317,#8318,#8319));
#2640=EDGE_LOOP('',(#8320,#8321,#8322,#8323,#8324,#8325));
#2641=EDGE_LOOP('',(#8326,#8327,#8328,#8329,#8330));
#2642=EDGE_LOOP('',(#8331,#8332,#8333,#8334));
#2643=EDGE_LOOP('',(#8335,#8336,#8337,#8338,#8339));
#2644=EDGE_LOOP('',(#8340,#8341,#8342,#8343));
#2645=EDGE_LOOP('',(#8344,#8345,#8346,#8347,#8348));
#2646=EDGE_LOOP('',(#8349,#8350,#8351));
#2647=EDGE_LOOP('',(#8352,#8353,#8354));
#2648=EDGE_LOOP('',(#8355,#8356,#8357));
#2649=EDGE_LOOP('',(#8358,#8359,#8360));
#2650=EDGE_LOOP('',(#8361,#8362,#8363,#8364,#8365,#8366));
#2651=EDGE_LOOP('',(#8367,#8368,#8369,#8370,#8371,#8372));
#2652=EDGE_LOOP('',(#8373,#8374,#8375,#8376));
#2653=EDGE_LOOP('',(#8377));
#2654=EDGE_LOOP('',(#8378,#8379,#8380,#8381,#8382,#8383));
#2655=EDGE_LOOP('',(#8384,#8385,#8386,#8387));
#2656=EDGE_LOOP('',(#8388,#8389,#8390,#8391,#8392,#8393));
#2657=EDGE_LOOP('',(#8394,#8395,#8396,#8397));
#2658=EDGE_LOOP('',(#8398,#8399,#8400,#8401));
#2659=EDGE_LOOP('',(#8402,#8403,#8404,#8405));
#2660=EDGE_LOOP('',(#8406));
#2661=EDGE_LOOP('',(#8407,#8408,#8409,#8410));
#3272=LINE('',#16344,#3977);
#3273=LINE('',#16346,#3978);
#3274=LINE('',#16348,#3979);
#3275=LINE('',#16350,#3980);
#3276=LINE('',#16352,#3981);
#3277=LINE('',#16353,#3982);
#3278=LINE('',#16356,#3983);
#3279=LINE('',#16360,#3984);
#3280=LINE('',#16363,#3985);
#3281=LINE('',#16368,#3986);
#3282=LINE('',#16370,#3987);
#3283=LINE('',#16371,#3988);
#3284=LINE('',#16374,#3989);
#3285=LINE('',#16376,#3990);
#3286=LINE('',#16378,#3991);
#3287=LINE('',#16380,#3992);
#3288=LINE('',#16381,#3993);
#3289=LINE('',#16384,#3994);
#3290=LINE('',#16386,#3995);
#3291=LINE('',#16388,#3996);
#3292=LINE('',#16390,#3997);
#3293=LINE('',#16391,#3998);
#3294=LINE('',#16394,#3999);
#3295=LINE('',#16396,#4000);
#3296=LINE('',#16397,#4001);
#3297=LINE('',#16400,#4002);
#3298=LINE('',#16402,#4003);
#3299=LINE('',#16404,#4004);
#3300=LINE('',#16405,#4005);
#3301=LINE('',#16408,#4006);
#3302=LINE('',#16410,#4007);
#3303=LINE('',#16411,#4008);
#3304=LINE('',#16412,#4009);
#3305=LINE('',#16415,#4010);
#3306=LINE('',#16417,#4011);
#3307=LINE('',#16419,#4012);
#3308=LINE('',#16420,#4013);
#3309=LINE('',#16423,#4014);
#3310=LINE('',#16424,#4015);
#3311=LINE('',#16427,#4016);
#3312=LINE('',#16429,#4017);
#3313=LINE('',#16431,#4018);
#3314=LINE('',#16433,#4019);
#3315=LINE('',#16434,#4020);
#3316=LINE('',#16437,#4021);
#3317=LINE('',#16439,#4022);
#3318=LINE('',#16441,#4023);
#3319=LINE('',#16443,#4024);
#3320=LINE('',#16444,#4025);
#3321=LINE('',#16447,#4026);
#3322=LINE('',#16449,#4027);
#3323=LINE('',#16450,#4028);
#3324=LINE('',#16455,#4029);
#3325=LINE('',#16457,#4030);
#3326=LINE('',#16459,#4031);
#3327=LINE('',#16460,#4032);
#3328=LINE('',#16463,#4033);
#3329=LINE('',#16464,#4034);
#3330=LINE('',#16465,#4035);
#3331=LINE('',#16468,#4036);
#3332=LINE('',#16470,#4037);
#3333=LINE('',#16472,#4038);
#3334=LINE('',#16473,#4039);
#3335=LINE('',#16476,#4040);
#3336=LINE('',#16477,#4041);
#3337=LINE('',#16480,#4042);
#3338=LINE('',#16482,#4043);
#3339=LINE('',#16484,#4044);
#3340=LINE('',#16486,#4045);
#3341=LINE('',#16487,#4046);
#3342=LINE('',#16490,#4047);
#3343=LINE('',#16491,#4048);
#3344=LINE('',#16494,#4049);
#3345=LINE('',#16496,#4050);
#3346=LINE('',#16498,#4051);
#3347=LINE('',#16499,#4052);
#3348=LINE('',#16502,#4053);
#3349=LINE('',#16504,#4054);
#3350=LINE('',#16506,#4055);
#3351=LINE('',#16507,#4056);
#3352=LINE('',#16511,#4057);
#3353=LINE('',#16513,#4058);
#3354=LINE('',#16515,#4059);
#3355=LINE('',#16517,#4060);
#3356=LINE('',#16519,#4061);
#3357=LINE('',#16520,#4062);
#3358=LINE('',#16523,#4063);
#3359=LINE('',#16525,#4064);
#3360=LINE('',#16526,#4065);
#3361=LINE('',#16528,#4066);
#3362=LINE('',#16529,#4067);
#3363=LINE('',#16532,#4068);
#3364=LINE('',#16534,#4069);
#3365=LINE('',#16536,#4070);
#3366=LINE('',#16537,#4071);
#3367=LINE('',#16540,#4072);
#3368=LINE('',#16541,#4073);
#3369=LINE('',#16547,#4074);
#3370=LINE('',#16548,#4075);
#3371=LINE('',#16550,#4076);
#3372=LINE('',#16551,#4077);
#3373=LINE('',#16553,#4078);
#3374=LINE('',#16556,#4079);
#3375=LINE('',#16558,#4080);
#3376=LINE('',#16560,#4081);
#3377=LINE('',#16561,#4082);
#3378=LINE('',#16564,#4083);
#3379=LINE('',#16565,#4084);
#3380=LINE('',#16566,#4085);
#3381=LINE('',#16570,#4086);
#3382=LINE('',#16572,#4087);
#3383=LINE('',#16573,#4088);
#3384=LINE('',#16574,#4089);
#3385=LINE('',#16577,#4090);
#3386=LINE('',#16579,#4091);
#3387=LINE('',#16581,#4092);
#3388=LINE('',#16583,#4093);
#3389=LINE('',#16584,#4094);
#3390=LINE('',#16587,#4095);
#3391=LINE('',#16589,#4096);
#3392=LINE('',#16591,#4097);
#3393=LINE('',#16593,#4098);
#3394=LINE('',#16594,#4099);
#3395=LINE('',#16597,#4100);
#3396=LINE('',#16599,#4101);
#3397=LINE('',#16600,#4102);
#3398=LINE('',#16603,#4103);
#3399=LINE('',#16605,#4104);
#3400=LINE('',#16607,#4105);
#3401=LINE('',#16608,#4106);
#3402=LINE('',#16611,#4107);
#3403=LINE('',#16613,#4108);
#3404=LINE('',#16614,#4109);
#3405=LINE('',#16615,#4110);
#3406=LINE('',#16618,#4111);
#3407=LINE('',#16620,#4112);
#3408=LINE('',#16622,#4113);
#3409=LINE('',#16623,#4114);
#3410=LINE('',#16626,#4115);
#3411=LINE('',#16627,#4116);
#3412=LINE('',#16630,#4117);
#3413=LINE('',#16632,#4118);
#3414=LINE('',#16634,#4119);
#3415=LINE('',#16636,#4120);
#3416=LINE('',#16637,#4121);
#3417=LINE('',#16640,#4122);
#3418=LINE('',#16642,#4123);
#3419=LINE('',#16644,#4124);
#3420=LINE('',#16646,#4125);
#3421=LINE('',#16647,#4126);
#3422=LINE('',#16650,#4127);
#3423=LINE('',#16654,#4128);
#3424=LINE('',#16657,#4129);
#3425=LINE('',#16662,#4130);
#3426=LINE('',#16664,#4131);
#3427=LINE('',#16665,#4132);
#3428=LINE('',#16668,#4133);
#3429=LINE('',#16669,#4134);
#3430=LINE('',#16670,#4135);
#3431=LINE('',#16673,#4136);
#3432=LINE('',#16675,#4137);
#3433=LINE('',#16676,#4138);
#3434=LINE('',#16679,#4139);
#3435=LINE('',#16681,#4140);
#3436=LINE('',#16682,#4141);
#3437=LINE('',#16755,#4142);
#3438=LINE('',#16782,#4143);
#3439=LINE('',#16784,#4144);
#3440=LINE('',#16786,#4145);
#3441=LINE('',#16788,#4146);
#3442=LINE('',#16789,#4147);
#3443=LINE('',#16814,#4148);
#3444=LINE('',#16820,#4149);
#3445=LINE('',#16822,#4150);
#3446=LINE('',#16823,#4151);
#3447=LINE('',#16826,#4152);
#3448=LINE('',#16827,#4153);
#3449=LINE('',#16830,#4154);
#3450=LINE('',#16878,#4155);
#3451=LINE('',#16880,#4156);
#3452=LINE('',#16881,#4157);
#3453=LINE('',#16884,#4158);
#3454=LINE('',#16886,#4159);
#3455=LINE('',#16887,#4160);
#3456=LINE('',#16959,#4161);
#3457=LINE('',#16986,#4162);
#3458=LINE('',#16988,#4163);
#3459=LINE('',#16990,#4164);
#3460=LINE('',#16992,#4165);
#3461=LINE('',#16993,#4166);
#3462=LINE('',#17018,#4167);
#3463=LINE('',#17024,#4168);
#3464=LINE('',#17027,#4169);
#3465=LINE('',#17028,#4170);
#3466=LINE('',#17029,#4171);
#3467=LINE('',#17031,#4172);
#3468=LINE('',#17034,#4173);
#3469=LINE('',#17035,#4174);
#3470=LINE('',#17037,#4175);
#3471=LINE('',#17039,#4176);
#3472=LINE('',#17087,#4177);
#3473=LINE('',#17092,#4178);
#3474=LINE('',#17094,#4179);
#3475=LINE('',#17097,#4180);
#3476=LINE('',#17102,#4181);
#3477=LINE('',#17104,#4182);
#3478=LINE('',#17107,#4183);
#3479=LINE('',#17112,#4184);
#3480=LINE('',#17114,#4185);
#3481=LINE('',#17117,#4186);
#3482=LINE('',#17122,#4187);
#3483=LINE('',#17124,#4188);
#3484=LINE('',#17129,#4189);
#3485=LINE('',#17133,#4190);
#3486=LINE('',#17140,#4191);
#3487=LINE('',#17147,#4192);
#3488=LINE('',#17151,#4193);
#3489=LINE('',#17155,#4194);
#3490=LINE('',#17159,#4195);
#3491=LINE('',#17166,#4196);
#3492=LINE('',#17173,#4197);
#3493=LINE('',#17176,#4198);
#3494=LINE('',#17179,#4199);
#3495=LINE('',#17183,#4200);
#3496=LINE('',#17190,#4201);
#3497=LINE('',#17197,#4202);
#3498=LINE('',#17200,#4203);
#3499=LINE('',#17354,#4204);
#3500=LINE('',#17426,#4205);
#3501=LINE('',#17543,#4206);
#3502=LINE('',#17547,#4207);
#3503=LINE('',#17549,#4208);
#3504=LINE('',#17551,#4209);
#3977=VECTOR('',#13626,1.);
#3978=VECTOR('',#13627,1.);
#3979=VECTOR('',#13628,1.);
#3980=VECTOR('',#13629,1.);
#3981=VECTOR('',#13630,1.);
#3982=VECTOR('',#13631,1.);
#3983=VECTOR('',#13634,1.);
#3984=VECTOR('',#13637,1.);
#3985=VECTOR('',#13640,1.);
#3986=VECTOR('',#13645,1.);
#3987=VECTOR('',#13646,1.);
#3988=VECTOR('',#13647,1.);
#3989=VECTOR('',#13650,1.);
#3990=VECTOR('',#13651,1.);
#3991=VECTOR('',#13652,1.);
#3992=VECTOR('',#13653,1.);
#3993=VECTOR('',#13654,1.);
#3994=VECTOR('',#13657,1.);
#3995=VECTOR('',#13658,1.);
#3996=VECTOR('',#13659,1.);
#3997=VECTOR('',#13660,1.);
#3998=VECTOR('',#13661,1.);
#3999=VECTOR('',#13664,1.);
#4000=VECTOR('',#13665,1.);
#4001=VECTOR('',#13666,1.);
#4002=VECTOR('',#13669,1.);
#4003=VECTOR('',#13670,1.);
#4004=VECTOR('',#13671,1.);
#4005=VECTOR('',#13672,1.);
#4006=VECTOR('',#13675,1.);
#4007=VECTOR('',#13676,1.);
#4008=VECTOR('',#13677,1.);
#4009=VECTOR('',#13678,1.);
#4010=VECTOR('',#13681,1.);
#4011=VECTOR('',#13682,1.);
#4012=VECTOR('',#13683,1.);
#4013=VECTOR('',#13684,1.);
#4014=VECTOR('',#13687,1.);
#4015=VECTOR('',#13688,1.);
#4016=VECTOR('',#13691,1.);
#4017=VECTOR('',#13692,1.);
#4018=VECTOR('',#13693,1.);
#4019=VECTOR('',#13694,1.);
#4020=VECTOR('',#13695,1.);
#4021=VECTOR('',#13698,1.);
#4022=VECTOR('',#13699,1.);
#4023=VECTOR('',#13700,1.);
#4024=VECTOR('',#13701,1.);
#4025=VECTOR('',#13702,1.);
#4026=VECTOR('',#13705,1.);
#4027=VECTOR('',#13706,1.);
#4028=VECTOR('',#13707,1.);
#4029=VECTOR('',#13712,1.);
#4030=VECTOR('',#13713,1.);
#4031=VECTOR('',#13714,1.);
#4032=VECTOR('',#13715,1.);
#4033=VECTOR('',#13718,1.);
#4034=VECTOR('',#13719,1.);
#4035=VECTOR('',#13720,1.);
#4036=VECTOR('',#13723,1.);
#4037=VECTOR('',#13724,1.);
#4038=VECTOR('',#13725,1.);
#4039=VECTOR('',#13726,1.);
#4040=VECTOR('',#13729,1.);
#4041=VECTOR('',#13730,1.);
#4042=VECTOR('',#13733,1.);
#4043=VECTOR('',#13734,1.);
#4044=VECTOR('',#13735,1.);
#4045=VECTOR('',#13736,1.);
#4046=VECTOR('',#13737,1.);
#4047=VECTOR('',#13740,1.);
#4048=VECTOR('',#13741,1.);
#4049=VECTOR('',#13744,1.);
#4050=VECTOR('',#13745,1.);
#4051=VECTOR('',#13746,1.);
#4052=VECTOR('',#13747,1.);
#4053=VECTOR('',#13750,1.);
#4054=VECTOR('',#13751,1.);
#4055=VECTOR('',#13752,1.);
#4056=VECTOR('',#13753,1.);
#4057=VECTOR('',#13756,1.);
#4058=VECTOR('',#13757,1.);
#4059=VECTOR('',#13758,1.);
#4060=VECTOR('',#13759,1.);
#4061=VECTOR('',#13760,1.);
#4062=VECTOR('',#13761,1.);
#4063=VECTOR('',#13764,1.);
#4064=VECTOR('',#13765,1.);
#4065=VECTOR('',#13766,1.);
#4066=VECTOR('',#13767,1.);
#4067=VECTOR('',#13768,1.);
#4068=VECTOR('',#13771,1.);
#4069=VECTOR('',#13772,1.);
#4070=VECTOR('',#13773,1.);
#4071=VECTOR('',#13774,1.);
#4072=VECTOR('',#13777,1.);
#4073=VECTOR('',#13778,1.);
#4074=VECTOR('',#13783,1.);
#4075=VECTOR('',#13784,1.);
#4076=VECTOR('',#13785,1.);
#4077=VECTOR('',#13786,1.);
#4078=VECTOR('',#13789,1.);
#4079=VECTOR('',#13792,1.);
#4080=VECTOR('',#13793,1.);
#4081=VECTOR('',#13794,1.);
#4082=VECTOR('',#13795,1.);
#4083=VECTOR('',#13798,1.);
#4084=VECTOR('',#13799,1.);
#4085=VECTOR('',#13800,1.);
#4086=VECTOR('',#13803,1.);
#4087=VECTOR('',#13804,1.);
#4088=VECTOR('',#13805,1.);
#4089=VECTOR('',#13806,1.);
#4090=VECTOR('',#13809,1.);
#4091=VECTOR('',#13810,1.);
#4092=VECTOR('',#13811,1.);
#4093=VECTOR('',#13812,1.);
#4094=VECTOR('',#13813,1.);
#4095=VECTOR('',#13816,1.);
#4096=VECTOR('',#13817,1.);
#4097=VECTOR('',#13818,1.);
#4098=VECTOR('',#13819,1.);
#4099=VECTOR('',#13820,1.);
#4100=VECTOR('',#13823,1.);
#4101=VECTOR('',#13824,1.);
#4102=VECTOR('',#13825,1.);
#4103=VECTOR('',#13828,1.);
#4104=VECTOR('',#13829,1.);
#4105=VECTOR('',#13830,1.);
#4106=VECTOR('',#13831,1.);
#4107=VECTOR('',#13834,1.);
#4108=VECTOR('',#13835,1.);
#4109=VECTOR('',#13836,1.);
#4110=VECTOR('',#13837,1.);
#4111=VECTOR('',#13840,1.);
#4112=VECTOR('',#13841,1.);
#4113=VECTOR('',#13842,1.);
#4114=VECTOR('',#13843,1.);
#4115=VECTOR('',#13846,1.);
#4116=VECTOR('',#13847,1.);
#4117=VECTOR('',#13850,1.);
#4118=VECTOR('',#13851,1.);
#4119=VECTOR('',#13852,1.);
#4120=VECTOR('',#13853,1.);
#4121=VECTOR('',#13854,1.);
#4122=VECTOR('',#13857,1.);
#4123=VECTOR('',#13858,1.);
#4124=VECTOR('',#13859,1.);
#4125=VECTOR('',#13860,1.);
#4126=VECTOR('',#13861,1.);
#4127=VECTOR('',#13864,1.);
#4128=VECTOR('',#13867,1.);
#4129=VECTOR('',#13870,1.);
#4130=VECTOR('',#13875,1.);
#4131=VECTOR('',#13876,1.);
#4132=VECTOR('',#13877,1.);
#4133=VECTOR('',#13880,1.);
#4134=VECTOR('',#13881,1.);
#4135=VECTOR('',#13882,1.);
#4136=VECTOR('',#13885,1.);
#4137=VECTOR('',#13886,1.);
#4138=VECTOR('',#13887,1.);
#4139=VECTOR('',#13890,1.);
#4140=VECTOR('',#13891,1.);
#4141=VECTOR('',#13892,1.);
#4142=VECTOR('',#13895,1.);
#4143=VECTOR('',#13896,1.);
#4144=VECTOR('',#13897,1.);
#4145=VECTOR('',#13898,1.);
#4146=VECTOR('',#13899,1.);
#4147=VECTOR('',#13900,1.);
#4148=VECTOR('',#13909,1.);
#4149=VECTOR('',#13910,1.);
#4150=VECTOR('',#13913,1.);
#4151=VECTOR('',#13914,1.);
#4152=VECTOR('',#13919,1.);
#4153=VECTOR('',#13920,1.);
#4154=VECTOR('',#13925,1.);
#4155=VECTOR('',#13928,1.);
#4156=VECTOR('',#13929,1.);
#4157=VECTOR('',#13930,1.);
#4158=VECTOR('',#13933,1.);
#4159=VECTOR('',#13934,1.);
#4160=VECTOR('',#13935,1.);
#4161=VECTOR('',#13938,1.);
#4162=VECTOR('',#13939,1.);
#4163=VECTOR('',#13940,1.);
#4164=VECTOR('',#13941,1.);
#4165=VECTOR('',#13942,1.);
#4166=VECTOR('',#13943,1.);
#4167=VECTOR('',#13952,1.);
#4168=VECTOR('',#13953,1.);
#4169=VECTOR('',#13956,1.);
#4170=VECTOR('',#13957,1.);
#4171=VECTOR('',#13958,1.);
#4172=VECTOR('',#13961,1.);
#4173=VECTOR('',#13966,1.);
#4174=VECTOR('',#13967,1.);
#4175=VECTOR('',#13970,1.);
#4176=VECTOR('',#13973,1.);
#4177=VECTOR('',#13976,0.36);
#4178=VECTOR('',#13983,0.33);
#4179=VECTOR('',#13986,0.36);
#4180=VECTOR('',#13989,0.36);
#4181=VECTOR('',#13996,0.33);
#4182=VECTOR('',#13999,0.36);
#4183=VECTOR('',#14002,0.36);
#4184=VECTOR('',#14009,0.33);
#4185=VECTOR('',#14012,0.36);
#4186=VECTOR('',#14015,0.36);
#4187=VECTOR('',#14022,0.33);
#4188=VECTOR('',#14025,0.36);
#4189=VECTOR('',#14030,1.35);
#4190=VECTOR('',#14035,1.3);
#4191=VECTOR('',#14044,0.7);
#4192=VECTOR('',#14053,1.3);
#4193=VECTOR('',#14058,1.35);
#4194=VECTOR('',#14063,1.35);
#4195=VECTOR('',#14068,1.3);
#4196=VECTOR('',#14077,0.7);
#4197=VECTOR('',#14086,1.3);
#4198=VECTOR('',#14091,1.35);
#4199=VECTOR('',#14094,1.35);
#4200=VECTOR('',#14099,1.3);
#4201=VECTOR('',#14108,0.7);
#4202=VECTOR('',#14117,1.3);
#4203=VECTOR('',#14122,1.35);
#4204=VECTOR('',#14137,1.);
#4205=VECTOR('',#14138,1.);
#4206=VECTOR('',#14163,1.);
#4207=VECTOR('',#14170,1.);
#4208=VECTOR('',#14173,1.);
#4209=VECTOR('',#14176,1.);
#4682=VERTEX_POINT('',#16342);
#4683=VERTEX_POINT('',#16343);
#4684=VERTEX_POINT('',#16345);
#4685=VERTEX_POINT('',#16347);
#4686=VERTEX_POINT('',#16349);
#4687=VERTEX_POINT('',#16351);
#4688=VERTEX_POINT('',#16355);
#4689=VERTEX_POINT('',#16357);
#4690=VERTEX_POINT('',#16359);
#4691=VERTEX_POINT('',#16361);
#4692=VERTEX_POINT('',#16364);
#4693=VERTEX_POINT('',#16367);
#4694=VERTEX_POINT('',#16369);
#4695=VERTEX_POINT('',#16373);
#4696=VERTEX_POINT('',#16375);
#4697=VERTEX_POINT('',#16377);
#4698=VERTEX_POINT('',#16379);
#4699=VERTEX_POINT('',#16383);
#4700=VERTEX_POINT('',#16385);
#4701=VERTEX_POINT('',#16387);
#4702=VERTEX_POINT('',#16389);
#4703=VERTEX_POINT('',#16393);
#4704=VERTEX_POINT('',#16395);
#4705=VERTEX_POINT('',#16399);
#4706=VERTEX_POINT('',#16401);
#4707=VERTEX_POINT('',#16403);
#4708=VERTEX_POINT('',#16407);
#4709=VERTEX_POINT('',#16409);
#4710=VERTEX_POINT('',#16414);
#4711=VERTEX_POINT('',#16416);
#4712=VERTEX_POINT('',#16418);
#4713=VERTEX_POINT('',#16422);
#4714=VERTEX_POINT('',#16426);
#4715=VERTEX_POINT('',#16428);
#4716=VERTEX_POINT('',#16430);
#4717=VERTEX_POINT('',#16432);
#4718=VERTEX_POINT('',#16436);
#4719=VERTEX_POINT('',#16438);
#4720=VERTEX_POINT('',#16440);
#4721=VERTEX_POINT('',#16442);
#4722=VERTEX_POINT('',#16446);
#4723=VERTEX_POINT('',#16448);
#4724=VERTEX_POINT('',#16451);
#4725=VERTEX_POINT('',#16454);
#4726=VERTEX_POINT('',#16456);
#4727=VERTEX_POINT('',#16458);
#4728=VERTEX_POINT('',#16462);
#4729=VERTEX_POINT('',#16467);
#4730=VERTEX_POINT('',#16469);
#4731=VERTEX_POINT('',#16471);
#4732=VERTEX_POINT('',#16475);
#4733=VERTEX_POINT('',#16479);
#4734=VERTEX_POINT('',#16481);
#4735=VERTEX_POINT('',#16483);
#4736=VERTEX_POINT('',#16485);
#4737=VERTEX_POINT('',#16489);
#4738=VERTEX_POINT('',#16493);
#4739=VERTEX_POINT('',#16495);
#4740=VERTEX_POINT('',#16497);
#4741=VERTEX_POINT('',#16501);
#4742=VERTEX_POINT('',#16503);
#4743=VERTEX_POINT('',#16505);
#4744=VERTEX_POINT('',#16509);
#4745=VERTEX_POINT('',#16510);
#4746=VERTEX_POINT('',#16512);
#4747=VERTEX_POINT('',#16514);
#4748=VERTEX_POINT('',#16516);
#4749=VERTEX_POINT('',#16518);
#4750=VERTEX_POINT('',#16522);
#4751=VERTEX_POINT('',#16524);
#4752=VERTEX_POINT('',#16527);
#4753=VERTEX_POINT('',#16531);
#4754=VERTEX_POINT('',#16533);
#4755=VERTEX_POINT('',#16535);
#4756=VERTEX_POINT('',#16539);
#4757=VERTEX_POINT('',#16542);
#4758=VERTEX_POINT('',#16545);
#4759=VERTEX_POINT('',#16546);
#4760=VERTEX_POINT('',#16549);
#4761=VERTEX_POINT('',#16555);
#4762=VERTEX_POINT('',#16557);
#4763=VERTEX_POINT('',#16559);
#4764=VERTEX_POINT('',#16563);
#4765=VERTEX_POINT('',#16568);
#4766=VERTEX_POINT('',#16569);
#4767=VERTEX_POINT('',#16571);
#4768=VERTEX_POINT('',#16576);
#4769=VERTEX_POINT('',#16578);
#4770=VERTEX_POINT('',#16580);
#4771=VERTEX_POINT('',#16582);
#4772=VERTEX_POINT('',#16586);
#4773=VERTEX_POINT('',#16588);
#4774=VERTEX_POINT('',#16590);
#4775=VERTEX_POINT('',#16592);
#4776=VERTEX_POINT('',#16596);
#4777=VERTEX_POINT('',#16598);
#4778=VERTEX_POINT('',#16602);
#4779=VERTEX_POINT('',#16604);
#4780=VERTEX_POINT('',#16606);
#4781=VERTEX_POINT('',#16610);
#4782=VERTEX_POINT('',#16612);
#4783=VERTEX_POINT('',#16617);
#4784=VERTEX_POINT('',#16619);
#4785=VERTEX_POINT('',#16621);
#4786=VERTEX_POINT('',#16625);
#4787=VERTEX_POINT('',#16629);
#4788=VERTEX_POINT('',#16631);
#4789=VERTEX_POINT('',#16633);
#4790=VERTEX_POINT('',#16635);
#4791=VERTEX_POINT('',#16639);
#4792=VERTEX_POINT('',#16641);
#4793=VERTEX_POINT('',#16643);
#4794=VERTEX_POINT('',#16645);
#4795=VERTEX_POINT('',#16649);
#4796=VERTEX_POINT('',#16651);
#4797=VERTEX_POINT('',#16653);
#4798=VERTEX_POINT('',#16655);
#4799=VERTEX_POINT('',#16658);
#4800=VERTEX_POINT('',#16661);
#4801=VERTEX_POINT('',#16663);
#4802=VERTEX_POINT('',#16667);
#4803=VERTEX_POINT('',#16672);
#4804=VERTEX_POINT('',#16674);
#4805=VERTEX_POINT('',#16678);
#4806=VERTEX_POINT('',#16680);
#4807=VERTEX_POINT('',#16699);
#4808=VERTEX_POINT('',#16700);
#4809=VERTEX_POINT('',#16729);
#4810=VERTEX_POINT('',#16739);
#4811=VERTEX_POINT('',#16749);
#4812=VERTEX_POINT('',#16754);
#4813=VERTEX_POINT('',#16756);
#4814=VERTEX_POINT('',#16761);
#4815=VERTEX_POINT('',#16771);
#4816=VERTEX_POINT('',#16776);
#4817=VERTEX_POINT('',#16781);
#4818=VERTEX_POINT('',#16783);
#4819=VERTEX_POINT('',#16785);
#4820=VERTEX_POINT('',#16787);
#4821=VERTEX_POINT('',#16790);
#4822=VERTEX_POINT('',#16792);
#4823=VERTEX_POINT('',#16794);
#4824=VERTEX_POINT('',#16796);
#4825=VERTEX_POINT('',#16815);
#4826=VERTEX_POINT('',#16847);
#4827=VERTEX_POINT('',#16877);
#4828=VERTEX_POINT('',#16879);
#4829=VERTEX_POINT('',#16883);
#4830=VERTEX_POINT('',#16885);
#4831=VERTEX_POINT('',#16904);
#4832=VERTEX_POINT('',#16905);
#4833=VERTEX_POINT('',#16934);
#4834=VERTEX_POINT('',#16944);
#4835=VERTEX_POINT('',#16953);
#4836=VERTEX_POINT('',#16958);
#4837=VERTEX_POINT('',#16960);
#4838=VERTEX_POINT('',#16965);
#4839=VERTEX_POINT('',#16975);
#4840=VERTEX_POINT('',#16980);
#4841=VERTEX_POINT('',#16985);
#4842=VERTEX_POINT('',#16987);
#4843=VERTEX_POINT('',#16989);
#4844=VERTEX_POINT('',#16991);
#4845=VERTEX_POINT('',#16994);
#4846=VERTEX_POINT('',#16996);
#4847=VERTEX_POINT('',#16998);
#4848=VERTEX_POINT('',#17000);
#4849=VERTEX_POINT('',#17019);
#4850=VERTEX_POINT('',#17026);
#4851=VERTEX_POINT('',#17056);
#4852=VERTEX_POINT('',#17086);
#4853=VERTEX_POINT('',#17090);
#4854=VERTEX_POINT('',#17096);
#4855=VERTEX_POINT('',#17100);
#4856=VERTEX_POINT('',#17106);
#4857=VERTEX_POINT('',#17110);
#4858=VERTEX_POINT('',#17116);
#4859=VERTEX_POINT('',#17120);
#4860=VERTEX_POINT('',#17126);
#4861=VERTEX_POINT('',#17128);
#4862=VERTEX_POINT('',#17132);
#4863=VERTEX_POINT('',#17136);
#4864=VERTEX_POINT('',#17139);
#4865=VERTEX_POINT('',#17143);
#4866=VERTEX_POINT('',#17146);
#4867=VERTEX_POINT('',#17150);
#4868=VERTEX_POINT('',#17154);
#4869=VERTEX_POINT('',#17158);
#4870=VERTEX_POINT('',#17162);
#4871=VERTEX_POINT('',#17165);
#4872=VERTEX_POINT('',#17169);
#4873=VERTEX_POINT('',#17172);
#4874=VERTEX_POINT('',#17178);
#4875=VERTEX_POINT('',#17182);
#4876=VERTEX_POINT('',#17186);
#4877=VERTEX_POINT('',#17189);
#4878=VERTEX_POINT('',#17193);
#4879=VERTEX_POINT('',#17196);
#4880=VERTEX_POINT('',#17237);
#4881=VERTEX_POINT('',#17283);
#4882=VERTEX_POINT('',#17339);
#4883=VERTEX_POINT('',#17344);
#4884=VERTEX_POINT('',#17411);
#4885=VERTEX_POINT('',#17416);
#4886=VERTEX_POINT('',#17528);
#4887=VERTEX_POINT('',#17532);
#4888=VERTEX_POINT('',#17537);
#4889=VERTEX_POINT('',#17541);
#5888=EDGE_CURVE('',#4682,#4683,#3272,.T.);
#5889=EDGE_CURVE('',#4683,#4684,#3273,.T.);
#5890=EDGE_CURVE('',#4684,#4685,#3274,.T.);
#5891=EDGE_CURVE('',#4685,#4686,#3275,.T.);
#5892=EDGE_CURVE('',#4686,#4687,#3276,.T.);
#5893=EDGE_CURVE('',#4687,#4682,#3277,.T.);
#5894=EDGE_CURVE('',#4688,#4686,#3278,.T.);
#5895=EDGE_CURVE('',#4689,#4688,#1405,.T.);
#5896=EDGE_CURVE('',#4690,#4689,#3279,.T.);
#5897=EDGE_CURVE('',#4691,#4690,#1406,.T.);
#5898=EDGE_CURVE('',#4687,#4691,#3280,.T.);
#5899=EDGE_CURVE('',#4692,#4692,#1407,.T.);
#5900=EDGE_CURVE('',#4685,#4693,#3281,.T.);
#5901=EDGE_CURVE('',#4694,#4693,#3282,.T.);
#5902=EDGE_CURVE('',#4694,#4688,#3283,.T.);
#5903=EDGE_CURVE('',#4695,#4684,#3284,.T.);
#5904=EDGE_CURVE('',#4696,#4695,#3285,.T.);
#5905=EDGE_CURVE('',#4697,#4696,#3286,.T.);
#5906=EDGE_CURVE('',#4698,#4697,#3287,.T.);
#5907=EDGE_CURVE('',#4693,#4698,#3288,.T.);
#5908=EDGE_CURVE('',#4695,#4699,#3289,.T.);
#5909=EDGE_CURVE('',#4699,#4700,#3290,.T.);
#5910=EDGE_CURVE('',#4700,#4701,#3291,.T.);
#5911=EDGE_CURVE('',#4701,#4702,#3292,.T.);
#5912=EDGE_CURVE('',#4702,#4696,#3293,.T.);
#5913=EDGE_CURVE('',#4703,#4701,#3294,.T.);
#5914=EDGE_CURVE('',#4704,#4703,#3295,.T.);
#5915=EDGE_CURVE('',#4702,#4704,#3296,.T.);
#5916=EDGE_CURVE('',#4700,#4705,#3297,.T.);
#5917=EDGE_CURVE('',#4706,#4705,#3298,.T.);
#5918=EDGE_CURVE('',#4706,#4707,#3299,.T.);
#5919=EDGE_CURVE('',#4703,#4707,#3300,.T.);
#5920=EDGE_CURVE('',#4708,#4682,#3301,.T.);
#5921=EDGE_CURVE('',#4709,#4708,#3302,.T.);
#5922=EDGE_CURVE('',#4705,#4709,#3303,.T.);
#5923=EDGE_CURVE('',#4683,#4699,#3304,.T.);
#5924=EDGE_CURVE('',#4707,#4710,#3305,.T.);
#5925=EDGE_CURVE('',#4710,#4711,#3306,.T.);
#5926=EDGE_CURVE('',#4711,#4712,#3307,.T.);
#5927=EDGE_CURVE('',#4712,#4704,#3308,.T.);
#5928=EDGE_CURVE('',#4712,#4713,#3309,.T.);
#5929=EDGE_CURVE('',#4697,#4713,#3310,.T.);
#5930=EDGE_CURVE('',#4714,#4711,#3311,.T.);
#5931=EDGE_CURVE('',#4715,#4714,#3312,.T.);
#5932=EDGE_CURVE('',#4716,#4715,#3313,.T.);
#5933=EDGE_CURVE('',#4717,#4716,#3314,.T.);
#5934=EDGE_CURVE('',#4713,#4717,#3315,.T.);
#5935=EDGE_CURVE('',#4714,#4718,#3316,.T.);
#5936=EDGE_CURVE('',#4718,#4719,#3317,.T.);
#5937=EDGE_CURVE('',#4719,#4720,#3318,.T.);
#5938=EDGE_CURVE('',#4720,#4721,#3319,.T.);
#5939=EDGE_CURVE('',#4721,#4715,#3320,.T.);
#5940=EDGE_CURVE('',#4722,#4720,#3321,.T.);
#5941=EDGE_CURVE('',#4723,#4722,#3322,.T.);
#5942=EDGE_CURVE('',#4721,#4723,#3323,.T.);
#5943=EDGE_CURVE('',#4724,#4724,#1408,.T.);
#5944=EDGE_CURVE('',#4719,#4725,#3324,.T.);
#5945=EDGE_CURVE('',#4726,#4725,#3325,.T.);
#5946=EDGE_CURVE('',#4726,#4727,#3326,.T.);
#5947=EDGE_CURVE('',#4722,#4727,#3327,.T.);
#5948=EDGE_CURVE('',#4728,#4706,#3328,.T.);
#5949=EDGE_CURVE('',#4725,#4728,#3329,.T.);
#5950=EDGE_CURVE('',#4710,#4718,#3330,.T.);
#5951=EDGE_CURVE('',#4727,#4729,#3331,.T.);
#5952=EDGE_CURVE('',#4729,#4730,#3332,.T.);
#5953=EDGE_CURVE('',#4730,#4731,#3333,.T.);
#5954=EDGE_CURVE('',#4731,#4723,#3334,.T.);
#5955=EDGE_CURVE('',#4731,#4732,#3335,.T.);
#5956=EDGE_CURVE('',#4716,#4732,#3336,.T.);
#5957=EDGE_CURVE('',#4733,#4730,#3337,.T.);
#5958=EDGE_CURVE('',#4734,#4733,#3338,.T.);
#5959=EDGE_CURVE('',#4735,#4734,#3339,.T.);
#5960=EDGE_CURVE('',#4736,#4735,#3340,.T.);
#5961=EDGE_CURVE('',#4732,#4736,#3341,.T.);
#5962=EDGE_CURVE('',#4729,#4737,#3342,.T.);
#5963=EDGE_CURVE('',#4733,#4737,#3343,.T.);
#5964=EDGE_CURVE('',#4737,#4738,#3344,.T.);
#5965=EDGE_CURVE('',#4738,#4739,#3345,.T.);
#5966=EDGE_CURVE('',#4739,#4740,#3346,.T.);
#5967=EDGE_CURVE('',#4740,#4734,#3347,.T.);
#5968=EDGE_CURVE('',#4740,#4741,#3348,.T.);
#5969=EDGE_CURVE('',#4742,#4741,#3349,.T.);
#5970=EDGE_CURVE('',#4742,#4743,#3350,.T.);
#5971=EDGE_CURVE('',#4735,#4743,#3351,.T.);
#5972=EDGE_CURVE('',#4744,#4745,#3352,.T.);
#5973=EDGE_CURVE('',#4745,#4746,#3353,.T.);
#5974=EDGE_CURVE('',#4746,#4747,#3354,.T.);
#5975=EDGE_CURVE('',#4747,#4748,#3355,.T.);
#5976=EDGE_CURVE('',#4748,#4749,#3356,.T.);
#5977=EDGE_CURVE('',#4749,#4744,#3357,.T.);
#5978=EDGE_CURVE('',#4750,#4744,#3358,.T.);
#5979=EDGE_CURVE('',#4751,#4750,#3359,.T.);
#5980=EDGE_CURVE('',#4743,#4751,#3360,.T.);
#5981=EDGE_CURVE('',#4752,#4742,#3361,.T.);
#5982=EDGE_CURVE('',#4745,#4752,#3362,.T.);
#5983=EDGE_CURVE('',#4749,#4753,#3363,.T.);
#5984=EDGE_CURVE('',#4754,#4753,#3364,.T.);
#5985=EDGE_CURVE('',#4754,#4755,#3365,.T.);
#5986=EDGE_CURVE('',#4750,#4755,#3366,.T.);
#5987=EDGE_CURVE('',#4756,#4748,#3367,.T.);
#5988=EDGE_CURVE('',#4753,#4756,#3368,.T.);
#5989=EDGE_CURVE('',#4757,#4757,#1409,.T.);
#5990=EDGE_CURVE('',#4758,#4759,#3369,.T.);
#5991=EDGE_CURVE('',#4759,#4752,#3370,.T.);
#5992=EDGE_CURVE('',#4741,#4760,#3371,.T.);
#5993=EDGE_CURVE('',#4760,#4758,#3372,.T.);
#5994=EDGE_CURVE('',#4759,#4746,#3373,.T.);
#5995=EDGE_CURVE('',#4761,#4758,#3374,.T.);
#5996=EDGE_CURVE('',#4762,#4761,#3375,.T.);
#5997=EDGE_CURVE('',#4763,#4762,#3376,.T.);
#5998=EDGE_CURVE('',#4747,#4763,#3377,.T.);
#5999=EDGE_CURVE('',#4738,#4764,#3378,.T.);
#6000=EDGE_CURVE('',#4761,#4764,#3379,.T.);
#6001=EDGE_CURVE('',#4760,#4739,#3380,.T.);
#6002=EDGE_CURVE('',#4765,#4766,#3381,.T.);
#6003=EDGE_CURVE('',#4766,#4767,#3382,.T.);
#6004=EDGE_CURVE('',#4767,#4754,#3383,.T.);
#6005=EDGE_CURVE('',#4756,#4765,#3384,.T.);
#6006=EDGE_CURVE('',#4768,#4767,#3385,.T.);
#6007=EDGE_CURVE('',#4769,#4768,#3386,.T.);
#6008=EDGE_CURVE('',#4770,#4769,#3387,.T.);
#6009=EDGE_CURVE('',#4771,#4770,#3388,.T.);
#6010=EDGE_CURVE('',#4755,#4771,#3389,.T.);
#6011=EDGE_CURVE('',#4768,#4772,#3390,.T.);
#6012=EDGE_CURVE('',#4772,#4773,#3391,.T.);
#6013=EDGE_CURVE('',#4773,#4774,#3392,.T.);
#6014=EDGE_CURVE('',#4774,#4775,#3393,.T.);
#6015=EDGE_CURVE('',#4775,#4769,#3394,.T.);
#6016=EDGE_CURVE('',#4776,#4774,#3395,.T.);
#6017=EDGE_CURVE('',#4777,#4776,#3396,.T.);
#6018=EDGE_CURVE('',#4775,#4777,#3397,.T.);
#6019=EDGE_CURVE('',#4773,#4778,#3398,.T.);
#6020=EDGE_CURVE('',#4779,#4778,#3399,.T.);
#6021=EDGE_CURVE('',#4779,#4780,#3400,.T.);
#6022=EDGE_CURVE('',#4776,#4780,#3401,.T.);
#6023=EDGE_CURVE('',#4781,#4765,#3402,.T.);
#6024=EDGE_CURVE('',#4782,#4781,#3403,.T.);
#6025=EDGE_CURVE('',#4778,#4782,#3404,.T.);
#6026=EDGE_CURVE('',#4766,#4772,#3405,.T.);
#6027=EDGE_CURVE('',#4780,#4783,#3406,.T.);
#6028=EDGE_CURVE('',#4783,#4784,#3407,.T.);
#6029=EDGE_CURVE('',#4784,#4785,#3408,.T.);
#6030=EDGE_CURVE('',#4785,#4777,#3409,.T.);
#6031=EDGE_CURVE('',#4785,#4786,#3410,.T.);
#6032=EDGE_CURVE('',#4770,#4786,#3411,.T.);
#6033=EDGE_CURVE('',#4787,#4784,#3412,.T.);
#6034=EDGE_CURVE('',#4788,#4787,#3413,.T.);
#6035=EDGE_CURVE('',#4789,#4788,#3414,.T.);
#6036=EDGE_CURVE('',#4790,#4789,#3415,.T.);
#6037=EDGE_CURVE('',#4786,#4790,#3416,.T.);
#6038=EDGE_CURVE('',#4787,#4791,#3417,.T.);
#6039=EDGE_CURVE('',#4791,#4792,#3418,.T.);
#6040=EDGE_CURVE('',#4792,#4793,#3419,.T.);
#6041=EDGE_CURVE('',#4793,#4794,#3420,.T.);
#6042=EDGE_CURVE('',#4794,#4788,#3421,.T.);
#6043=EDGE_CURVE('',#4795,#4793,#3422,.T.);
#6044=EDGE_CURVE('',#4796,#4795,#1410,.T.);
#6045=EDGE_CURVE('',#4797,#4796,#3423,.T.);
#6046=EDGE_CURVE('',#4798,#4797,#1411,.T.);
#6047=EDGE_CURVE('',#4794,#4798,#3424,.T.);
#6048=EDGE_CURVE('',#4799,#4799,#1412,.T.);
#6049=EDGE_CURVE('',#4792,#4800,#3425,.T.);
#6050=EDGE_CURVE('',#4801,#4800,#3426,.T.);
#6051=EDGE_CURVE('',#4801,#4795,#3427,.T.);
#6052=EDGE_CURVE('',#4802,#4779,#3428,.T.);
#6053=EDGE_CURVE('',#4800,#4802,#3429,.T.);
#6054=EDGE_CURVE('',#4783,#4791,#3430,.T.);
#6055=EDGE_CURVE('',#4790,#4803,#3431,.T.);
#6056=EDGE_CURVE('',#4803,#4804,#3432,.T.);
#6057=EDGE_CURVE('',#4804,#4771,#3433,.T.);
#6058=EDGE_CURVE('',#4789,#4805,#3434,.T.);
#6059=EDGE_CURVE('',#4806,#4805,#3435,.T.);
#6060=EDGE_CURVE('',#4806,#4803,#3436,.T.);
#6061=EDGE_CURVE('',#4807,#4808,#457,.T.);
#6062=EDGE_CURVE('',#4808,#4806,#458,.T.);
#6063=EDGE_CURVE('',#4805,#4807,#459,.T.);
#6064=EDGE_CURVE('',#4807,#4809,#460,.T.);
#6065=EDGE_CURVE('',#4809,#4808,#461,.T.);
#6066=EDGE_CURVE('',#4810,#4809,#462,.T.);
#6067=EDGE_CURVE('',#4811,#4810,#463,.T.);
#6068=EDGE_CURVE('',#4812,#4811,#3437,.T.);
#6069=EDGE_CURVE('',#4813,#4812,#464,.T.);
#6070=EDGE_CURVE('',#4814,#4813,#465,.T.);
#6071=EDGE_CURVE('',#4815,#4814,#466,.T.);
#6072=EDGE_CURVE('',#4816,#4815,#467,.T.);
#6073=EDGE_CURVE('',#4817,#4816,#3438,.T.);
#6074=EDGE_CURVE('',#4818,#4817,#3439,.T.);
#6075=EDGE_CURVE('',#4819,#4818,#3440,.T.);
#6076=EDGE_CURVE('',#4820,#4819,#3441,.T.);
#6077=EDGE_CURVE('',#4804,#4820,#3442,.T.);
#6078=EDGE_CURVE('',#4821,#4821,#1413,.T.);
#6079=EDGE_CURVE('',#4822,#4822,#1414,.T.);
#6080=EDGE_CURVE('',#4823,#4823,#1415,.T.);
#6081=EDGE_CURVE('',#4824,#4824,#1416,.T.);
#6082=EDGE_CURVE('',#4798,#4805,#3443,.T.);
#6083=EDGE_CURVE('',#4798,#4825,#468,.T.);
#6084=EDGE_CURVE('',#4809,#4825,#3444,.T.);
#6085=EDGE_CURVE('',#4751,#4820,#3445,.T.);
#6086=EDGE_CURVE('',#4819,#4736,#3446,.T.);
#6087=EDGE_CURVE('',#4717,#4818,#3447,.T.);
#6088=EDGE_CURVE('',#4817,#4698,#3448,.T.);
#6089=EDGE_CURVE('',#4816,#4694,#3449,.T.);
#6090=EDGE_CURVE('',#4815,#4826,#469,.T.);
#6091=EDGE_CURVE('',#4826,#4694,#470,.T.);
#6092=EDGE_CURVE('',#4814,#4826,#471,.T.);
#6093=EDGE_CURVE('',#4709,#4827,#3450,.T.);
#6094=EDGE_CURVE('',#4827,#4828,#3451,.T.);
#6095=EDGE_CURVE('',#4828,#4728,#3452,.T.);
#6096=EDGE_CURVE('',#4708,#4829,#3453,.T.);
#6097=EDGE_CURVE('',#4830,#4829,#3454,.T.);
#6098=EDGE_CURVE('',#4830,#4827,#3455,.T.);
#6099=EDGE_CURVE('',#4831,#4832,#472,.T.);
#6100=EDGE_CURVE('',#4832,#4830,#473,.T.);
#6101=EDGE_CURVE('',#4829,#4831,#474,.T.);
#6102=EDGE_CURVE('',#4831,#4833,#475,.T.);
#6103=EDGE_CURVE('',#4833,#4832,#476,.T.);
#6104=EDGE_CURVE('',#4834,#4833,#477,.T.);
#6105=EDGE_CURVE('',#4835,#4834,#478,.T.);
#6106=EDGE_CURVE('',#4836,#4835,#3456,.T.);
#6107=EDGE_CURVE('',#4837,#4836,#479,.T.);
#6108=EDGE_CURVE('',#4838,#4837,#480,.T.);
#6109=EDGE_CURVE('',#4839,#4838,#481,.T.);
#6110=EDGE_CURVE('',#4840,#4839,#482,.T.);
#6111=EDGE_CURVE('',#4841,#4840,#3457,.T.);
#6112=EDGE_CURVE('',#4842,#4841,#3458,.T.);
#6113=EDGE_CURVE('',#4843,#4842,#3459,.T.);
#6114=EDGE_CURVE('',#4844,#4843,#3460,.T.);
#6115=EDGE_CURVE('',#4828,#4844,#3461,.T.);
#6116=EDGE_CURVE('',#4845,#4845,#1417,.T.);
#6117=EDGE_CURVE('',#4846,#4846,#1418,.T.);
#6118=EDGE_CURVE('',#4847,#4847,#1419,.T.);
#6119=EDGE_CURVE('',#4848,#4848,#1420,.T.);
#6120=EDGE_CURVE('',#4691,#4829,#3462,.T.);
#6121=EDGE_CURVE('',#4691,#4849,#483,.T.);
#6122=EDGE_CURVE('',#4833,#4849,#3463,.T.);
#6123=EDGE_CURVE('',#4764,#4850,#3464,.T.);
#6124=EDGE_CURVE('',#4850,#4844,#3465,.T.);
#6125=EDGE_CURVE('',#4843,#4762,#3466,.T.);
#6126=EDGE_CURVE('',#4850,#4726,#3467,.T.);
#6127=EDGE_CURVE('',#4782,#4842,#3468,.T.);
#6128=EDGE_CURVE('',#4841,#4802,#3469,.T.);
#6129=EDGE_CURVE('',#4781,#4763,#3470,.T.);
#6130=EDGE_CURVE('',#4840,#4801,#3471,.T.);
#6131=EDGE_CURVE('',#4839,#4851,#484,.T.);
#6132=EDGE_CURVE('',#4851,#4801,#485,.T.);
#6133=EDGE_CURVE('',#4838,#4851,#486,.T.);
#6134=EDGE_CURVE('',#4848,#4852,#3472,.T.);
#6135=EDGE_CURVE('',#4852,#4852,#1421,.T.);
#6136=EDGE_CURVE('',#4853,#4853,#1422,.T.);
#6137=EDGE_CURVE('',#4853,#4852,#3473,.T.);
#6138=EDGE_CURVE('',#4824,#4853,#3474,.T.);
#6139=EDGE_CURVE('',#4845,#4854,#3475,.T.);
#6140=EDGE_CURVE('',#4854,#4854,#1423,.T.);
#6141=EDGE_CURVE('',#4855,#4855,#1424,.T.);
#6142=EDGE_CURVE('',#4855,#4854,#3476,.T.);
#6143=EDGE_CURVE('',#4821,#4855,#3477,.T.);
#6144=EDGE_CURVE('',#4847,#4856,#3478,.T.);
#6145=EDGE_CURVE('',#4856,#4856,#1425,.T.);
#6146=EDGE_CURVE('',#4857,#4857,#1426,.T.);
#6147=EDGE_CURVE('',#4857,#4856,#3479,.T.);
#6148=EDGE_CURVE('',#4823,#4857,#3480,.T.);
#6149=EDGE_CURVE('',#4846,#4858,#3481,.T.);
#6150=EDGE_CURVE('',#4858,#4858,#1427,.T.);
#6151=EDGE_CURVE('',#4859,#4859,#1428,.T.);
#6152=EDGE_CURVE('',#4859,#4858,#3482,.T.);
#6153=EDGE_CURVE('',#4822,#4859,#3483,.T.);
#6154=EDGE_CURVE('',#4860,#4860,#1429,.T.);
#6155=EDGE_CURVE('',#4860,#4861,#3484,.T.);
#6156=EDGE_CURVE('',#4861,#4861,#1430,.T.);
#6157=EDGE_CURVE('',#4861,#4862,#3485,.T.);
#6158=EDGE_CURVE('',#4862,#4862,#1431,.T.);
#6159=EDGE_CURVE('',#4863,#4863,#1432,.T.);
#6160=EDGE_CURVE('',#4863,#4864,#3486,.T.);
#6161=EDGE_CURVE('',#4864,#4864,#1433,.T.);
#6162=EDGE_CURVE('',#4865,#4865,#1434,.T.);
#6163=EDGE_CURVE('',#4865,#4866,#3487,.T.);
#6164=EDGE_CURVE('',#4866,#4866,#1435,.T.);
#6165=EDGE_CURVE('',#4866,#4867,#3488,.T.);
#6166=EDGE_CURVE('',#4867,#4867,#1436,.T.);
#6167=EDGE_CURVE('',#4799,#4868,#3489,.T.);
#6168=EDGE_CURVE('',#4868,#4868,#1437,.T.);
#6169=EDGE_CURVE('',#4868,#4869,#3490,.T.);
#6170=EDGE_CURVE('',#4869,#4869,#1438,.T.);
#6171=EDGE_CURVE('',#4870,#4870,#1439,.T.);
#6172=EDGE_CURVE('',#4870,#4871,#3491,.T.);
#6173=EDGE_CURVE('',#4871,#4871,#1440,.T.);
#6174=EDGE_CURVE('',#4872,#4872,#1441,.T.);
#6175=EDGE_CURVE('',#4872,#4873,#3492,.T.);
#6176=EDGE_CURVE('',#4873,#4873,#1442,.T.);
#6177=EDGE_CURVE('',#4873,#4757,#3493,.T.);
#6178=EDGE_CURVE('',#4724,#4874,#3494,.T.);
#6179=EDGE_CURVE('',#4874,#4874,#1443,.T.);
#6180=EDGE_CURVE('',#4874,#4875,#3495,.T.);
#6181=EDGE_CURVE('',#4875,#4875,#1444,.T.);
#6182=EDGE_CURVE('',#4876,#4876,#1445,.T.);
#6183=EDGE_CURVE('',#4876,#4877,#3496,.T.);
#6184=EDGE_CURVE('',#4877,#4877,#1446,.T.);
#6185=EDGE_CURVE('',#4878,#4878,#1447,.T.);
#6186=EDGE_CURVE('',#4878,#4879,#3497,.T.);
#6187=EDGE_CURVE('',#4879,#4879,#1448,.T.);
#6188=EDGE_CURVE('',#4879,#4692,#3498,.T.);
#6189=EDGE_CURVE('',#4880,#4810,#487,.T.);
#6190=EDGE_CURVE('',#4825,#4880,#488,.T.);
#6191=EDGE_CURVE('',#4881,#4834,#489,.T.);
#6192=EDGE_CURVE('',#4849,#4881,#490,.T.);
#6193=EDGE_CURVE('',#4813,#4882,#491,.T.);
#6194=EDGE_CURVE('',#4882,#4883,#492,.T.);
#6195=EDGE_CURVE('',#4883,#4814,#3499,.T.);
#6196=EDGE_CURVE('',#4883,#4688,#493,.T.);
#6197=EDGE_CURVE('',#4837,#4884,#494,.T.);
#6198=EDGE_CURVE('',#4884,#4885,#495,.T.);
#6199=EDGE_CURVE('',#4885,#4838,#3500,.T.);
#6200=EDGE_CURVE('',#4885,#4795,#496,.T.);
#6201=EDGE_CURVE('',#4880,#4811,#497,.T.);
#6202=EDGE_CURVE('',#4881,#4835,#498,.T.);
#6203=EDGE_CURVE('',#4812,#4882,#499,.T.);
#6204=EDGE_CURVE('',#4836,#4884,#500,.T.);
#6205=EDGE_CURVE('',#4797,#4886,#1449,.T.);
#6206=EDGE_CURVE('',#4886,#4811,#1450,.T.);
#6207=EDGE_CURVE('',#4836,#4887,#1451,.T.);
#6208=EDGE_CURVE('',#4796,#4887,#1452,.T.);
#6209=EDGE_CURVE('',#4690,#4888,#1453,.T.);
#6210=EDGE_CURVE('',#4888,#4835,#1454,.T.);
#6211=EDGE_CURVE('',#4689,#4889,#1455,.T.);
#6212=EDGE_CURVE('',#4889,#4888,#3501,.T.);
#6213=EDGE_CURVE('',#4812,#4889,#1456,.T.);
#6214=EDGE_CURVE('',#4887,#4886,#3502,.T.);
#6215=EDGE_CURVE('',#4888,#4887,#3503,.T.);
#6216=EDGE_CURVE('',#4886,#4889,#3504,.T.);
#7753=ORIENTED_EDGE('',*,*,#5888,.T.);
#7754=ORIENTED_EDGE('',*,*,#5889,.T.);
#7755=ORIENTED_EDGE('',*,*,#5890,.T.);
#7756=ORIENTED_EDGE('',*,*,#5891,.T.);
#7757=ORIENTED_EDGE('',*,*,#5892,.T.);
#7758=ORIENTED_EDGE('',*,*,#5893,.T.);
#7759=ORIENTED_EDGE('',*,*,#5892,.F.);
#7760=ORIENTED_EDGE('',*,*,#5894,.F.);
#7761=ORIENTED_EDGE('',*,*,#5895,.F.);
#7762=ORIENTED_EDGE('',*,*,#5896,.F.);
#7763=ORIENTED_EDGE('',*,*,#5897,.F.);
#7764=ORIENTED_EDGE('',*,*,#5898,.F.);
#7765=ORIENTED_EDGE('',*,*,#5899,.T.);
#7766=ORIENTED_EDGE('',*,*,#5891,.F.);
#7767=ORIENTED_EDGE('',*,*,#5900,.T.);
#7768=ORIENTED_EDGE('',*,*,#5901,.F.);
#7769=ORIENTED_EDGE('',*,*,#5902,.T.);
#7770=ORIENTED_EDGE('',*,*,#5894,.T.);
#7771=ORIENTED_EDGE('',*,*,#5890,.F.);
#7772=ORIENTED_EDGE('',*,*,#5903,.F.);
#7773=ORIENTED_EDGE('',*,*,#5904,.F.);
#7774=ORIENTED_EDGE('',*,*,#5905,.F.);
#7775=ORIENTED_EDGE('',*,*,#5906,.F.);
#7776=ORIENTED_EDGE('',*,*,#5907,.F.);
#7777=ORIENTED_EDGE('',*,*,#5900,.F.);
#7778=ORIENTED_EDGE('',*,*,#5904,.T.);
#7779=ORIENTED_EDGE('',*,*,#5908,.T.);
#7780=ORIENTED_EDGE('',*,*,#5909,.T.);
#7781=ORIENTED_EDGE('',*,*,#5910,.T.);
#7782=ORIENTED_EDGE('',*,*,#5911,.T.);
#7783=ORIENTED_EDGE('',*,*,#5912,.T.);
#7784=ORIENTED_EDGE('',*,*,#5911,.F.);
#7785=ORIENTED_EDGE('',*,*,#5913,.F.);
#7786=ORIENTED_EDGE('',*,*,#5914,.F.);
#7787=ORIENTED_EDGE('',*,*,#5915,.F.);
#7788=ORIENTED_EDGE('',*,*,#5910,.F.);
#7789=ORIENTED_EDGE('',*,*,#5916,.T.);
#7790=ORIENTED_EDGE('',*,*,#5917,.F.);
#7791=ORIENTED_EDGE('',*,*,#5918,.T.);
#7792=ORIENTED_EDGE('',*,*,#5919,.F.);
#7793=ORIENTED_EDGE('',*,*,#5913,.T.);
#7794=ORIENTED_EDGE('',*,*,#5888,.F.);
#7795=ORIENTED_EDGE('',*,*,#5920,.F.);
#7796=ORIENTED_EDGE('',*,*,#5921,.F.);
#7797=ORIENTED_EDGE('',*,*,#5922,.F.);
#7798=ORIENTED_EDGE('',*,*,#5916,.F.);
#7799=ORIENTED_EDGE('',*,*,#5909,.F.);
#7800=ORIENTED_EDGE('',*,*,#5923,.F.);
#7801=ORIENTED_EDGE('',*,*,#5924,.T.);
#7802=ORIENTED_EDGE('',*,*,#5925,.T.);
#7803=ORIENTED_EDGE('',*,*,#5926,.T.);
#7804=ORIENTED_EDGE('',*,*,#5927,.T.);
#7805=ORIENTED_EDGE('',*,*,#5914,.T.);
#7806=ORIENTED_EDGE('',*,*,#5919,.T.);
#7807=ORIENTED_EDGE('',*,*,#5912,.F.);
#7808=ORIENTED_EDGE('',*,*,#5915,.T.);
#7809=ORIENTED_EDGE('',*,*,#5927,.F.);
#7810=ORIENTED_EDGE('',*,*,#5928,.T.);
#7811=ORIENTED_EDGE('',*,*,#5929,.F.);
#7812=ORIENTED_EDGE('',*,*,#5905,.T.);
#7813=ORIENTED_EDGE('',*,*,#5926,.F.);
#7814=ORIENTED_EDGE('',*,*,#5930,.F.);
#7815=ORIENTED_EDGE('',*,*,#5931,.F.);
#7816=ORIENTED_EDGE('',*,*,#5932,.F.);
#7817=ORIENTED_EDGE('',*,*,#5933,.F.);
#7818=ORIENTED_EDGE('',*,*,#5934,.F.);
#7819=ORIENTED_EDGE('',*,*,#5928,.F.);
#7820=ORIENTED_EDGE('',*,*,#5931,.T.);
#7821=ORIENTED_EDGE('',*,*,#5935,.T.);
#7822=ORIENTED_EDGE('',*,*,#5936,.T.);
#7823=ORIENTED_EDGE('',*,*,#5937,.T.);
#7824=ORIENTED_EDGE('',*,*,#5938,.T.);
#7825=ORIENTED_EDGE('',*,*,#5939,.T.);
#7826=ORIENTED_EDGE('',*,*,#5938,.F.);
#7827=ORIENTED_EDGE('',*,*,#5940,.F.);
#7828=ORIENTED_EDGE('',*,*,#5941,.F.);
#7829=ORIENTED_EDGE('',*,*,#5942,.F.);
#7830=ORIENTED_EDGE('',*,*,#5943,.T.);
#7831=ORIENTED_EDGE('',*,*,#5937,.F.);
#7832=ORIENTED_EDGE('',*,*,#5944,.T.);
#7833=ORIENTED_EDGE('',*,*,#5945,.F.);
#7834=ORIENTED_EDGE('',*,*,#5946,.T.);
#7835=ORIENTED_EDGE('',*,*,#5947,.F.);
#7836=ORIENTED_EDGE('',*,*,#5940,.T.);
#7837=ORIENTED_EDGE('',*,*,#5924,.F.);
#7838=ORIENTED_EDGE('',*,*,#5918,.F.);
#7839=ORIENTED_EDGE('',*,*,#5948,.F.);
#7840=ORIENTED_EDGE('',*,*,#5949,.F.);
#7841=ORIENTED_EDGE('',*,*,#5944,.F.);
#7842=ORIENTED_EDGE('',*,*,#5936,.F.);
#7843=ORIENTED_EDGE('',*,*,#5950,.F.);
#7844=ORIENTED_EDGE('',*,*,#5951,.T.);
#7845=ORIENTED_EDGE('',*,*,#5952,.T.);
#7846=ORIENTED_EDGE('',*,*,#5953,.T.);
#7847=ORIENTED_EDGE('',*,*,#5954,.T.);
#7848=ORIENTED_EDGE('',*,*,#5941,.T.);
#7849=ORIENTED_EDGE('',*,*,#5947,.T.);
#7850=ORIENTED_EDGE('',*,*,#5939,.F.);
#7851=ORIENTED_EDGE('',*,*,#5942,.T.);
#7852=ORIENTED_EDGE('',*,*,#5954,.F.);
#7853=ORIENTED_EDGE('',*,*,#5955,.T.);
#7854=ORIENTED_EDGE('',*,*,#5956,.F.);
#7855=ORIENTED_EDGE('',*,*,#5932,.T.);
#7856=ORIENTED_EDGE('',*,*,#5953,.F.);
#7857=ORIENTED_EDGE('',*,*,#5957,.F.);
#7858=ORIENTED_EDGE('',*,*,#5958,.F.);
#7859=ORIENTED_EDGE('',*,*,#5959,.F.);
#7860=ORIENTED_EDGE('',*,*,#5960,.F.);
#7861=ORIENTED_EDGE('',*,*,#5961,.F.);
#7862=ORIENTED_EDGE('',*,*,#5955,.F.);
#7863=ORIENTED_EDGE('',*,*,#5952,.F.);
#7864=ORIENTED_EDGE('',*,*,#5962,.T.);
#7865=ORIENTED_EDGE('',*,*,#5963,.F.);
#7866=ORIENTED_EDGE('',*,*,#5957,.T.);
#7867=ORIENTED_EDGE('',*,*,#5958,.T.);
#7868=ORIENTED_EDGE('',*,*,#5963,.T.);
#7869=ORIENTED_EDGE('',*,*,#5964,.T.);
#7870=ORIENTED_EDGE('',*,*,#5965,.T.);
#7871=ORIENTED_EDGE('',*,*,#5966,.T.);
#7872=ORIENTED_EDGE('',*,*,#5967,.T.);
#7873=ORIENTED_EDGE('',*,*,#5967,.F.);
#7874=ORIENTED_EDGE('',*,*,#5968,.T.);
#7875=ORIENTED_EDGE('',*,*,#5969,.F.);
#7876=ORIENTED_EDGE('',*,*,#5970,.T.);
#7877=ORIENTED_EDGE('',*,*,#5971,.F.);
#7878=ORIENTED_EDGE('',*,*,#5959,.T.);
#7879=ORIENTED_EDGE('',*,*,#5972,.T.);
#7880=ORIENTED_EDGE('',*,*,#5973,.T.);
#7881=ORIENTED_EDGE('',*,*,#5974,.T.);
#7882=ORIENTED_EDGE('',*,*,#5975,.T.);
#7883=ORIENTED_EDGE('',*,*,#5976,.T.);
#7884=ORIENTED_EDGE('',*,*,#5977,.T.);
#7885=ORIENTED_EDGE('',*,*,#5972,.F.);
#7886=ORIENTED_EDGE('',*,*,#5978,.F.);
#7887=ORIENTED_EDGE('',*,*,#5979,.F.);
#7888=ORIENTED_EDGE('',*,*,#5980,.F.);
#7889=ORIENTED_EDGE('',*,*,#5970,.F.);
#7890=ORIENTED_EDGE('',*,*,#5981,.F.);
#7891=ORIENTED_EDGE('',*,*,#5982,.F.);
#7892=ORIENTED_EDGE('',*,*,#5977,.F.);
#7893=ORIENTED_EDGE('',*,*,#5983,.T.);
#7894=ORIENTED_EDGE('',*,*,#5984,.F.);
#7895=ORIENTED_EDGE('',*,*,#5985,.T.);
#7896=ORIENTED_EDGE('',*,*,#5986,.F.);
#7897=ORIENTED_EDGE('',*,*,#5978,.T.);
#7898=ORIENTED_EDGE('',*,*,#5976,.F.);
#7899=ORIENTED_EDGE('',*,*,#5987,.F.);
#7900=ORIENTED_EDGE('',*,*,#5988,.F.);
#7901=ORIENTED_EDGE('',*,*,#5983,.F.);
#7902=ORIENTED_EDGE('',*,*,#5989,.T.);
#7903=ORIENTED_EDGE('',*,*,#5990,.T.);
#7904=ORIENTED_EDGE('',*,*,#5991,.T.);
#7905=ORIENTED_EDGE('',*,*,#5981,.T.);
#7906=ORIENTED_EDGE('',*,*,#5969,.T.);
#7907=ORIENTED_EDGE('',*,*,#5992,.T.);
#7908=ORIENTED_EDGE('',*,*,#5993,.T.);
#7909=ORIENTED_EDGE('',*,*,#5973,.F.);
#7910=ORIENTED_EDGE('',*,*,#5982,.T.);
#7911=ORIENTED_EDGE('',*,*,#5991,.F.);
#7912=ORIENTED_EDGE('',*,*,#5994,.T.);
#7913=ORIENTED_EDGE('',*,*,#5974,.F.);
#7914=ORIENTED_EDGE('',*,*,#5994,.F.);
#7915=ORIENTED_EDGE('',*,*,#5990,.F.);
#7916=ORIENTED_EDGE('',*,*,#5995,.F.);
#7917=ORIENTED_EDGE('',*,*,#5996,.F.);
#7918=ORIENTED_EDGE('',*,*,#5997,.F.);
#7919=ORIENTED_EDGE('',*,*,#5998,.F.);
#7920=ORIENTED_EDGE('',*,*,#5965,.F.);
#7921=ORIENTED_EDGE('',*,*,#5999,.T.);
#7922=ORIENTED_EDGE('',*,*,#6000,.F.);
#7923=ORIENTED_EDGE('',*,*,#5995,.T.);
#7924=ORIENTED_EDGE('',*,*,#5993,.F.);
#7925=ORIENTED_EDGE('',*,*,#6001,.T.);
#7926=ORIENTED_EDGE('',*,*,#6002,.T.);
#7927=ORIENTED_EDGE('',*,*,#6003,.T.);
#7928=ORIENTED_EDGE('',*,*,#6004,.T.);
#7929=ORIENTED_EDGE('',*,*,#5984,.T.);
#7930=ORIENTED_EDGE('',*,*,#5988,.T.);
#7931=ORIENTED_EDGE('',*,*,#6005,.T.);
#7932=ORIENTED_EDGE('',*,*,#6004,.F.);
#7933=ORIENTED_EDGE('',*,*,#6006,.F.);
#7934=ORIENTED_EDGE('',*,*,#6007,.F.);
#7935=ORIENTED_EDGE('',*,*,#6008,.F.);
#7936=ORIENTED_EDGE('',*,*,#6009,.F.);
#7937=ORIENTED_EDGE('',*,*,#6010,.F.);
#7938=ORIENTED_EDGE('',*,*,#5985,.F.);
#7939=ORIENTED_EDGE('',*,*,#6007,.T.);
#7940=ORIENTED_EDGE('',*,*,#6011,.T.);
#7941=ORIENTED_EDGE('',*,*,#6012,.T.);
#7942=ORIENTED_EDGE('',*,*,#6013,.T.);
#7943=ORIENTED_EDGE('',*,*,#6014,.T.);
#7944=ORIENTED_EDGE('',*,*,#6015,.T.);
#7945=ORIENTED_EDGE('',*,*,#6014,.F.);
#7946=ORIENTED_EDGE('',*,*,#6016,.F.);
#7947=ORIENTED_EDGE('',*,*,#6017,.F.);
#7948=ORIENTED_EDGE('',*,*,#6018,.F.);
#7949=ORIENTED_EDGE('',*,*,#6013,.F.);
#7950=ORIENTED_EDGE('',*,*,#6019,.T.);
#7951=ORIENTED_EDGE('',*,*,#6020,.F.);
#7952=ORIENTED_EDGE('',*,*,#6021,.T.);
#7953=ORIENTED_EDGE('',*,*,#6022,.F.);
#7954=ORIENTED_EDGE('',*,*,#6016,.T.);
#7955=ORIENTED_EDGE('',*,*,#6002,.F.);
#7956=ORIENTED_EDGE('',*,*,#6023,.F.);
#7957=ORIENTED_EDGE('',*,*,#6024,.F.);
#7958=ORIENTED_EDGE('',*,*,#6025,.F.);
#7959=ORIENTED_EDGE('',*,*,#6019,.F.);
#7960=ORIENTED_EDGE('',*,*,#6012,.F.);
#7961=ORIENTED_EDGE('',*,*,#6026,.F.);
#7962=ORIENTED_EDGE('',*,*,#6027,.T.);
#7963=ORIENTED_EDGE('',*,*,#6028,.T.);
#7964=ORIENTED_EDGE('',*,*,#6029,.T.);
#7965=ORIENTED_EDGE('',*,*,#6030,.T.);
#7966=ORIENTED_EDGE('',*,*,#6017,.T.);
#7967=ORIENTED_EDGE('',*,*,#6022,.T.);
#7968=ORIENTED_EDGE('',*,*,#6015,.F.);
#7969=ORIENTED_EDGE('',*,*,#6018,.T.);
#7970=ORIENTED_EDGE('',*,*,#6030,.F.);
#7971=ORIENTED_EDGE('',*,*,#6031,.T.);
#7972=ORIENTED_EDGE('',*,*,#6032,.F.);
#7973=ORIENTED_EDGE('',*,*,#6008,.T.);
#7974=ORIENTED_EDGE('',*,*,#6029,.F.);
#7975=ORIENTED_EDGE('',*,*,#6033,.F.);
#7976=ORIENTED_EDGE('',*,*,#6034,.F.);
#7977=ORIENTED_EDGE('',*,*,#6035,.F.);
#7978=ORIENTED_EDGE('',*,*,#6036,.F.);
#7979=ORIENTED_EDGE('',*,*,#6037,.F.);
#7980=ORIENTED_EDGE('',*,*,#6031,.F.);
#7981=ORIENTED_EDGE('',*,*,#6034,.T.);
#7982=ORIENTED_EDGE('',*,*,#6038,.T.);
#7983=ORIENTED_EDGE('',*,*,#6039,.T.);
#7984=ORIENTED_EDGE('',*,*,#6040,.T.);
#7985=ORIENTED_EDGE('',*,*,#6041,.T.);
#7986=ORIENTED_EDGE('',*,*,#6042,.T.);
#7987=ORIENTED_EDGE('',*,*,#6041,.F.);
#7988=ORIENTED_EDGE('',*,*,#6043,.F.);
#7989=ORIENTED_EDGE('',*,*,#6044,.F.);
#7990=ORIENTED_EDGE('',*,*,#6045,.F.);
#7991=ORIENTED_EDGE('',*,*,#6046,.F.);
#7992=ORIENTED_EDGE('',*,*,#6047,.F.);
#7993=ORIENTED_EDGE('',*,*,#6048,.T.);
#7994=ORIENTED_EDGE('',*,*,#6040,.F.);
#7995=ORIENTED_EDGE('',*,*,#6049,.T.);
#7996=ORIENTED_EDGE('',*,*,#6050,.F.);
#7997=ORIENTED_EDGE('',*,*,#6051,.T.);
#7998=ORIENTED_EDGE('',*,*,#6043,.T.);
#7999=ORIENTED_EDGE('',*,*,#6027,.F.);
#8000=ORIENTED_EDGE('',*,*,#6021,.F.);
#8001=ORIENTED_EDGE('',*,*,#6052,.F.);
#8002=ORIENTED_EDGE('',*,*,#6053,.F.);
#8003=ORIENTED_EDGE('',*,*,#6049,.F.);
#8004=ORIENTED_EDGE('',*,*,#6039,.F.);
#8005=ORIENTED_EDGE('',*,*,#6054,.F.);
#8006=ORIENTED_EDGE('',*,*,#6009,.T.);
#8007=ORIENTED_EDGE('',*,*,#6032,.T.);
#8008=ORIENTED_EDGE('',*,*,#6037,.T.);
#8009=ORIENTED_EDGE('',*,*,#6055,.T.);
#8010=ORIENTED_EDGE('',*,*,#6056,.T.);
#8011=ORIENTED_EDGE('',*,*,#6057,.T.);
#8012=ORIENTED_EDGE('',*,*,#6055,.F.);
#8013=ORIENTED_EDGE('',*,*,#6036,.T.);
#8014=ORIENTED_EDGE('',*,*,#6058,.T.);
#8015=ORIENTED_EDGE('',*,*,#6059,.F.);
#8016=ORIENTED_EDGE('',*,*,#6060,.T.);
#8017=ORIENTED_EDGE('',*,*,#6061,.T.);
#8018=ORIENTED_EDGE('',*,*,#6062,.T.);
#8019=ORIENTED_EDGE('',*,*,#6059,.T.);
#8020=ORIENTED_EDGE('',*,*,#6063,.T.);
#8021=ORIENTED_EDGE('',*,*,#6061,.F.);
#8022=ORIENTED_EDGE('',*,*,#6064,.T.);
#8023=ORIENTED_EDGE('',*,*,#6065,.T.);
#8024=ORIENTED_EDGE('',*,*,#6056,.F.);
#8025=ORIENTED_EDGE('',*,*,#6060,.F.);
#8026=ORIENTED_EDGE('',*,*,#6062,.F.);
#8027=ORIENTED_EDGE('',*,*,#6065,.F.);
#8028=ORIENTED_EDGE('',*,*,#6066,.F.);
#8029=ORIENTED_EDGE('',*,*,#6067,.F.);
#8030=ORIENTED_EDGE('',*,*,#6068,.F.);
#8031=ORIENTED_EDGE('',*,*,#6069,.F.);
#8032=ORIENTED_EDGE('',*,*,#6070,.F.);
#8033=ORIENTED_EDGE('',*,*,#6071,.F.);
#8034=ORIENTED_EDGE('',*,*,#6072,.F.);
#8035=ORIENTED_EDGE('',*,*,#6073,.F.);
#8036=ORIENTED_EDGE('',*,*,#6074,.F.);
#8037=ORIENTED_EDGE('',*,*,#6075,.F.);
#8038=ORIENTED_EDGE('',*,*,#6076,.F.);
#8039=ORIENTED_EDGE('',*,*,#6077,.F.);
#8040=ORIENTED_EDGE('',*,*,#6078,.F.);
#8041=ORIENTED_EDGE('',*,*,#6079,.F.);
#8042=ORIENTED_EDGE('',*,*,#6080,.F.);
#8043=ORIENTED_EDGE('',*,*,#6081,.F.);
#8044=ORIENTED_EDGE('',*,*,#6064,.F.);
#8045=ORIENTED_EDGE('',*,*,#6063,.F.);
#8046=ORIENTED_EDGE('',*,*,#6082,.F.);
#8047=ORIENTED_EDGE('',*,*,#6083,.T.);
#8048=ORIENTED_EDGE('',*,*,#6084,.F.);
#8049=ORIENTED_EDGE('',*,*,#5960,.T.);
#8050=ORIENTED_EDGE('',*,*,#5971,.T.);
#8051=ORIENTED_EDGE('',*,*,#5980,.T.);
#8052=ORIENTED_EDGE('',*,*,#6085,.T.);
#8053=ORIENTED_EDGE('',*,*,#6076,.T.);
#8054=ORIENTED_EDGE('',*,*,#6086,.T.);
#8055=ORIENTED_EDGE('',*,*,#6057,.F.);
#8056=ORIENTED_EDGE('',*,*,#6077,.T.);
#8057=ORIENTED_EDGE('',*,*,#6085,.F.);
#8058=ORIENTED_EDGE('',*,*,#5979,.T.);
#8059=ORIENTED_EDGE('',*,*,#5986,.T.);
#8060=ORIENTED_EDGE('',*,*,#6010,.T.);
#8061=ORIENTED_EDGE('',*,*,#6087,.T.);
#8062=ORIENTED_EDGE('',*,*,#6074,.T.);
#8063=ORIENTED_EDGE('',*,*,#6088,.T.);
#8064=ORIENTED_EDGE('',*,*,#5906,.T.);
#8065=ORIENTED_EDGE('',*,*,#5929,.T.);
#8066=ORIENTED_EDGE('',*,*,#5934,.T.);
#8067=ORIENTED_EDGE('',*,*,#6086,.F.);
#8068=ORIENTED_EDGE('',*,*,#6075,.T.);
#8069=ORIENTED_EDGE('',*,*,#6087,.F.);
#8070=ORIENTED_EDGE('',*,*,#5933,.T.);
#8071=ORIENTED_EDGE('',*,*,#5956,.T.);
#8072=ORIENTED_EDGE('',*,*,#5961,.T.);
#8073=ORIENTED_EDGE('',*,*,#6088,.F.);
#8074=ORIENTED_EDGE('',*,*,#6073,.T.);
#8075=ORIENTED_EDGE('',*,*,#6089,.T.);
#8076=ORIENTED_EDGE('',*,*,#5901,.T.);
#8077=ORIENTED_EDGE('',*,*,#5907,.T.);
#8078=ORIENTED_EDGE('',*,*,#6090,.T.);
#8079=ORIENTED_EDGE('',*,*,#6091,.T.);
#8080=ORIENTED_EDGE('',*,*,#6089,.F.);
#8081=ORIENTED_EDGE('',*,*,#6072,.T.);
#8082=ORIENTED_EDGE('',*,*,#6090,.F.);
#8083=ORIENTED_EDGE('',*,*,#6071,.T.);
#8084=ORIENTED_EDGE('',*,*,#6092,.T.);
#8085=ORIENTED_EDGE('',*,*,#5948,.T.);
#8086=ORIENTED_EDGE('',*,*,#5917,.T.);
#8087=ORIENTED_EDGE('',*,*,#5922,.T.);
#8088=ORIENTED_EDGE('',*,*,#6093,.T.);
#8089=ORIENTED_EDGE('',*,*,#6094,.T.);
#8090=ORIENTED_EDGE('',*,*,#6095,.T.);
#8091=ORIENTED_EDGE('',*,*,#6093,.F.);
#8092=ORIENTED_EDGE('',*,*,#5921,.T.);
#8093=ORIENTED_EDGE('',*,*,#6096,.T.);
#8094=ORIENTED_EDGE('',*,*,#6097,.F.);
#8095=ORIENTED_EDGE('',*,*,#6098,.T.);
#8096=ORIENTED_EDGE('',*,*,#6099,.T.);
#8097=ORIENTED_EDGE('',*,*,#6100,.T.);
#8098=ORIENTED_EDGE('',*,*,#6097,.T.);
#8099=ORIENTED_EDGE('',*,*,#6101,.T.);
#8100=ORIENTED_EDGE('',*,*,#6099,.F.);
#8101=ORIENTED_EDGE('',*,*,#6102,.T.);
#8102=ORIENTED_EDGE('',*,*,#6103,.T.);
#8103=ORIENTED_EDGE('',*,*,#6094,.F.);
#8104=ORIENTED_EDGE('',*,*,#6098,.F.);
#8105=ORIENTED_EDGE('',*,*,#6100,.F.);
#8106=ORIENTED_EDGE('',*,*,#6103,.F.);
#8107=ORIENTED_EDGE('',*,*,#6104,.F.);
#8108=ORIENTED_EDGE('',*,*,#6105,.F.);
#8109=ORIENTED_EDGE('',*,*,#6106,.F.);
#8110=ORIENTED_EDGE('',*,*,#6107,.F.);
#8111=ORIENTED_EDGE('',*,*,#6108,.F.);
#8112=ORIENTED_EDGE('',*,*,#6109,.F.);
#8113=ORIENTED_EDGE('',*,*,#6110,.F.);
#8114=ORIENTED_EDGE('',*,*,#6111,.F.);
#8115=ORIENTED_EDGE('',*,*,#6112,.F.);
#8116=ORIENTED_EDGE('',*,*,#6113,.F.);
#8117=ORIENTED_EDGE('',*,*,#6114,.F.);
#8118=ORIENTED_EDGE('',*,*,#6115,.F.);
#8119=ORIENTED_EDGE('',*,*,#6116,.F.);
#8120=ORIENTED_EDGE('',*,*,#6117,.F.);
#8121=ORIENTED_EDGE('',*,*,#6118,.F.);
#8122=ORIENTED_EDGE('',*,*,#6119,.F.);
#8123=ORIENTED_EDGE('',*,*,#6102,.F.);
#8124=ORIENTED_EDGE('',*,*,#6101,.F.);
#8125=ORIENTED_EDGE('',*,*,#6120,.F.);
#8126=ORIENTED_EDGE('',*,*,#6121,.T.);
#8127=ORIENTED_EDGE('',*,*,#6122,.F.);
#8128=ORIENTED_EDGE('',*,*,#5996,.T.);
#8129=ORIENTED_EDGE('',*,*,#6000,.T.);
#8130=ORIENTED_EDGE('',*,*,#6123,.T.);
#8131=ORIENTED_EDGE('',*,*,#6124,.T.);
#8132=ORIENTED_EDGE('',*,*,#6114,.T.);
#8133=ORIENTED_EDGE('',*,*,#6125,.T.);
#8134=ORIENTED_EDGE('',*,*,#6095,.F.);
#8135=ORIENTED_EDGE('',*,*,#6115,.T.);
#8136=ORIENTED_EDGE('',*,*,#6124,.F.);
#8137=ORIENTED_EDGE('',*,*,#6126,.T.);
#8138=ORIENTED_EDGE('',*,*,#5945,.T.);
#8139=ORIENTED_EDGE('',*,*,#5949,.T.);
#8140=ORIENTED_EDGE('',*,*,#5951,.F.);
#8141=ORIENTED_EDGE('',*,*,#5946,.F.);
#8142=ORIENTED_EDGE('',*,*,#6126,.F.);
#8143=ORIENTED_EDGE('',*,*,#6123,.F.);
#8144=ORIENTED_EDGE('',*,*,#5999,.F.);
#8145=ORIENTED_EDGE('',*,*,#5964,.F.);
#8146=ORIENTED_EDGE('',*,*,#5962,.F.);
#8147=ORIENTED_EDGE('',*,*,#6127,.T.);
#8148=ORIENTED_EDGE('',*,*,#6112,.T.);
#8149=ORIENTED_EDGE('',*,*,#6128,.T.);
#8150=ORIENTED_EDGE('',*,*,#6052,.T.);
#8151=ORIENTED_EDGE('',*,*,#6020,.T.);
#8152=ORIENTED_EDGE('',*,*,#6025,.T.);
#8153=ORIENTED_EDGE('',*,*,#6125,.F.);
#8154=ORIENTED_EDGE('',*,*,#6113,.T.);
#8155=ORIENTED_EDGE('',*,*,#6127,.F.);
#8156=ORIENTED_EDGE('',*,*,#6024,.T.);
#8157=ORIENTED_EDGE('',*,*,#6129,.T.);
#8158=ORIENTED_EDGE('',*,*,#5997,.T.);
#8159=ORIENTED_EDGE('',*,*,#6128,.F.);
#8160=ORIENTED_EDGE('',*,*,#6111,.T.);
#8161=ORIENTED_EDGE('',*,*,#6130,.T.);
#8162=ORIENTED_EDGE('',*,*,#6050,.T.);
#8163=ORIENTED_EDGE('',*,*,#6053,.T.);
#8164=ORIENTED_EDGE('',*,*,#6131,.T.);
#8165=ORIENTED_EDGE('',*,*,#6132,.T.);
#8166=ORIENTED_EDGE('',*,*,#6130,.F.);
#8167=ORIENTED_EDGE('',*,*,#6110,.T.);
#8168=ORIENTED_EDGE('',*,*,#6131,.F.);
#8169=ORIENTED_EDGE('',*,*,#6109,.T.);
#8170=ORIENTED_EDGE('',*,*,#6133,.T.);
#8171=ORIENTED_EDGE('',*,*,#6119,.T.);
#8172=ORIENTED_EDGE('',*,*,#6134,.T.);
#8173=ORIENTED_EDGE('',*,*,#6135,.T.);
#8174=ORIENTED_EDGE('',*,*,#6134,.F.);
#8175=ORIENTED_EDGE('',*,*,#6136,.F.);
#8176=ORIENTED_EDGE('',*,*,#6137,.T.);
#8177=ORIENTED_EDGE('',*,*,#6135,.F.);
#8178=ORIENTED_EDGE('',*,*,#6137,.F.);
#8179=ORIENTED_EDGE('',*,*,#6081,.T.);
#8180=ORIENTED_EDGE('',*,*,#6138,.T.);
#8181=ORIENTED_EDGE('',*,*,#6136,.T.);
#8182=ORIENTED_EDGE('',*,*,#6138,.F.);
#8183=ORIENTED_EDGE('',*,*,#6116,.T.);
#8184=ORIENTED_EDGE('',*,*,#6139,.T.);
#8185=ORIENTED_EDGE('',*,*,#6140,.T.);
#8186=ORIENTED_EDGE('',*,*,#6139,.F.);
#8187=ORIENTED_EDGE('',*,*,#6141,.F.);
#8188=ORIENTED_EDGE('',*,*,#6142,.T.);
#8189=ORIENTED_EDGE('',*,*,#6140,.F.);
#8190=ORIENTED_EDGE('',*,*,#6142,.F.);
#8191=ORIENTED_EDGE('',*,*,#6078,.T.);
#8192=ORIENTED_EDGE('',*,*,#6143,.T.);
#8193=ORIENTED_EDGE('',*,*,#6141,.T.);
#8194=ORIENTED_EDGE('',*,*,#6143,.F.);
#8195=ORIENTED_EDGE('',*,*,#6118,.T.);
#8196=ORIENTED_EDGE('',*,*,#6144,.T.);
#8197=ORIENTED_EDGE('',*,*,#6145,.T.);
#8198=ORIENTED_EDGE('',*,*,#6144,.F.);
#8199=ORIENTED_EDGE('',*,*,#6146,.F.);
#8200=ORIENTED_EDGE('',*,*,#6147,.T.);
#8201=ORIENTED_EDGE('',*,*,#6145,.F.);
#8202=ORIENTED_EDGE('',*,*,#6147,.F.);
#8203=ORIENTED_EDGE('',*,*,#6080,.T.);
#8204=ORIENTED_EDGE('',*,*,#6148,.T.);
#8205=ORIENTED_EDGE('',*,*,#6146,.T.);
#8206=ORIENTED_EDGE('',*,*,#6148,.F.);
#8207=ORIENTED_EDGE('',*,*,#6117,.T.);
#8208=ORIENTED_EDGE('',*,*,#6149,.T.);
#8209=ORIENTED_EDGE('',*,*,#6150,.T.);
#8210=ORIENTED_EDGE('',*,*,#6149,.F.);
#8211=ORIENTED_EDGE('',*,*,#6151,.F.);
#8212=ORIENTED_EDGE('',*,*,#6152,.T.);
#8213=ORIENTED_EDGE('',*,*,#6150,.F.);
#8214=ORIENTED_EDGE('',*,*,#6152,.F.);
#8215=ORIENTED_EDGE('',*,*,#6079,.T.);
#8216=ORIENTED_EDGE('',*,*,#6153,.T.);
#8217=ORIENTED_EDGE('',*,*,#6151,.T.);
#8218=ORIENTED_EDGE('',*,*,#6153,.F.);
#8219=ORIENTED_EDGE('',*,*,#6154,.F.);
#8220=ORIENTED_EDGE('',*,*,#6155,.T.);
#8221=ORIENTED_EDGE('',*,*,#6156,.T.);
#8222=ORIENTED_EDGE('',*,*,#6155,.F.);
#8223=ORIENTED_EDGE('',*,*,#6156,.F.);
#8224=ORIENTED_EDGE('',*,*,#6157,.T.);
#8225=ORIENTED_EDGE('',*,*,#6158,.T.);
#8226=ORIENTED_EDGE('',*,*,#6157,.F.);
#8227=ORIENTED_EDGE('',*,*,#6158,.F.);
#8228=ORIENTED_EDGE('',*,*,#6159,.T.);
#8229=ORIENTED_EDGE('',*,*,#6159,.F.);
#8230=ORIENTED_EDGE('',*,*,#6160,.T.);
#8231=ORIENTED_EDGE('',*,*,#6161,.T.);
#8232=ORIENTED_EDGE('',*,*,#6160,.F.);
#8233=ORIENTED_EDGE('',*,*,#6162,.T.);
#8234=ORIENTED_EDGE('',*,*,#6161,.F.);
#8235=ORIENTED_EDGE('',*,*,#6162,.F.);
#8236=ORIENTED_EDGE('',*,*,#6163,.T.);
#8237=ORIENTED_EDGE('',*,*,#6164,.T.);
#8238=ORIENTED_EDGE('',*,*,#6163,.F.);
#8239=ORIENTED_EDGE('',*,*,#6164,.F.);
#8240=ORIENTED_EDGE('',*,*,#6165,.T.);
#8241=ORIENTED_EDGE('',*,*,#6166,.F.);
#8242=ORIENTED_EDGE('',*,*,#6165,.F.);
#8243=ORIENTED_EDGE('',*,*,#6048,.F.);
#8244=ORIENTED_EDGE('',*,*,#6167,.T.);
#8245=ORIENTED_EDGE('',*,*,#6168,.T.);
#8246=ORIENTED_EDGE('',*,*,#6167,.F.);
#8247=ORIENTED_EDGE('',*,*,#6168,.F.);
#8248=ORIENTED_EDGE('',*,*,#6169,.T.);
#8249=ORIENTED_EDGE('',*,*,#6170,.T.);
#8250=ORIENTED_EDGE('',*,*,#6169,.F.);
#8251=ORIENTED_EDGE('',*,*,#6170,.F.);
#8252=ORIENTED_EDGE('',*,*,#6171,.T.);
#8253=ORIENTED_EDGE('',*,*,#6171,.F.);
#8254=ORIENTED_EDGE('',*,*,#6172,.T.);
#8255=ORIENTED_EDGE('',*,*,#6173,.T.);
#8256=ORIENTED_EDGE('',*,*,#6172,.F.);
#8257=ORIENTED_EDGE('',*,*,#6174,.T.);
#8258=ORIENTED_EDGE('',*,*,#6173,.F.);
#8259=ORIENTED_EDGE('',*,*,#6174,.F.);
#8260=ORIENTED_EDGE('',*,*,#6175,.T.);
#8261=ORIENTED_EDGE('',*,*,#6176,.T.);
#8262=ORIENTED_EDGE('',*,*,#6175,.F.);
#8263=ORIENTED_EDGE('',*,*,#6176,.F.);
#8264=ORIENTED_EDGE('',*,*,#6177,.T.);
#8265=ORIENTED_EDGE('',*,*,#5989,.F.);
#8266=ORIENTED_EDGE('',*,*,#6177,.F.);
#8267=ORIENTED_EDGE('',*,*,#5943,.F.);
#8268=ORIENTED_EDGE('',*,*,#6178,.T.);
#8269=ORIENTED_EDGE('',*,*,#6179,.T.);
#8270=ORIENTED_EDGE('',*,*,#6178,.F.);
#8271=ORIENTED_EDGE('',*,*,#6179,.F.);
#8272=ORIENTED_EDGE('',*,*,#6180,.T.);
#8273=ORIENTED_EDGE('',*,*,#6181,.T.);
#8274=ORIENTED_EDGE('',*,*,#6180,.F.);
#8275=ORIENTED_EDGE('',*,*,#6181,.F.);
#8276=ORIENTED_EDGE('',*,*,#6182,.T.);
#8277=ORIENTED_EDGE('',*,*,#6182,.F.);
#8278=ORIENTED_EDGE('',*,*,#6183,.T.);
#8279=ORIENTED_EDGE('',*,*,#6184,.T.);
#8280=ORIENTED_EDGE('',*,*,#6183,.F.);
#8281=ORIENTED_EDGE('',*,*,#6185,.T.);
#8282=ORIENTED_EDGE('',*,*,#6184,.F.);
#8283=ORIENTED_EDGE('',*,*,#6185,.F.);
#8284=ORIENTED_EDGE('',*,*,#6186,.T.);
#8285=ORIENTED_EDGE('',*,*,#6187,.T.);
#8286=ORIENTED_EDGE('',*,*,#6186,.F.);
#8287=ORIENTED_EDGE('',*,*,#6187,.F.);
#8288=ORIENTED_EDGE('',*,*,#6188,.T.);
#8289=ORIENTED_EDGE('',*,*,#5899,.F.);
#8290=ORIENTED_EDGE('',*,*,#6188,.F.);
#8291=ORIENTED_EDGE('',*,*,#6189,.T.);
#8292=ORIENTED_EDGE('',*,*,#6066,.T.);
#8293=ORIENTED_EDGE('',*,*,#6084,.T.);
#8294=ORIENTED_EDGE('',*,*,#6190,.T.);
#8295=ORIENTED_EDGE('',*,*,#6191,.T.);
#8296=ORIENTED_EDGE('',*,*,#6104,.T.);
#8297=ORIENTED_EDGE('',*,*,#6122,.T.);
#8298=ORIENTED_EDGE('',*,*,#6192,.T.);
#8299=ORIENTED_EDGE('',*,*,#6028,.F.);
#8300=ORIENTED_EDGE('',*,*,#6054,.T.);
#8301=ORIENTED_EDGE('',*,*,#6038,.F.);
#8302=ORIENTED_EDGE('',*,*,#6033,.T.);
#8303=ORIENTED_EDGE('',*,*,#6003,.F.);
#8304=ORIENTED_EDGE('',*,*,#6026,.T.);
#8305=ORIENTED_EDGE('',*,*,#6011,.F.);
#8306=ORIENTED_EDGE('',*,*,#6006,.T.);
#8307=ORIENTED_EDGE('',*,*,#5925,.F.);
#8308=ORIENTED_EDGE('',*,*,#5950,.T.);
#8309=ORIENTED_EDGE('',*,*,#5935,.F.);
#8310=ORIENTED_EDGE('',*,*,#5930,.T.);
#8311=ORIENTED_EDGE('',*,*,#5889,.F.);
#8312=ORIENTED_EDGE('',*,*,#5923,.T.);
#8313=ORIENTED_EDGE('',*,*,#5908,.F.);
#8314=ORIENTED_EDGE('',*,*,#5903,.T.);
#8315=ORIENTED_EDGE('',*,*,#5893,.F.);
#8316=ORIENTED_EDGE('',*,*,#5898,.T.);
#8317=ORIENTED_EDGE('',*,*,#6120,.T.);
#8318=ORIENTED_EDGE('',*,*,#6096,.F.);
#8319=ORIENTED_EDGE('',*,*,#5920,.T.);
#8320=ORIENTED_EDGE('',*,*,#5975,.F.);
#8321=ORIENTED_EDGE('',*,*,#5998,.T.);
#8322=ORIENTED_EDGE('',*,*,#6129,.F.);
#8323=ORIENTED_EDGE('',*,*,#6023,.T.);
#8324=ORIENTED_EDGE('',*,*,#6005,.F.);
#8325=ORIENTED_EDGE('',*,*,#5987,.T.);
#8326=ORIENTED_EDGE('',*,*,#6042,.F.);
#8327=ORIENTED_EDGE('',*,*,#6047,.T.);
#8328=ORIENTED_EDGE('',*,*,#6082,.T.);
#8329=ORIENTED_EDGE('',*,*,#6058,.F.);
#8330=ORIENTED_EDGE('',*,*,#6035,.T.);
#8331=ORIENTED_EDGE('',*,*,#6193,.T.);
#8332=ORIENTED_EDGE('',*,*,#6194,.T.);
#8333=ORIENTED_EDGE('',*,*,#6195,.T.);
#8334=ORIENTED_EDGE('',*,*,#6070,.T.);
#8335=ORIENTED_EDGE('',*,*,#6092,.F.);
#8336=ORIENTED_EDGE('',*,*,#6195,.F.);
#8337=ORIENTED_EDGE('',*,*,#6196,.T.);
#8338=ORIENTED_EDGE('',*,*,#5902,.F.);
#8339=ORIENTED_EDGE('',*,*,#6091,.F.);
#8340=ORIENTED_EDGE('',*,*,#6197,.T.);
#8341=ORIENTED_EDGE('',*,*,#6198,.T.);
#8342=ORIENTED_EDGE('',*,*,#6199,.T.);
#8343=ORIENTED_EDGE('',*,*,#6108,.T.);
#8344=ORIENTED_EDGE('',*,*,#6133,.F.);
#8345=ORIENTED_EDGE('',*,*,#6199,.F.);
#8346=ORIENTED_EDGE('',*,*,#6200,.T.);
#8347=ORIENTED_EDGE('',*,*,#6051,.F.);
#8348=ORIENTED_EDGE('',*,*,#6132,.F.);
#8349=ORIENTED_EDGE('',*,*,#6189,.F.);
#8350=ORIENTED_EDGE('',*,*,#6201,.T.);
#8351=ORIENTED_EDGE('',*,*,#6067,.T.);
#8352=ORIENTED_EDGE('',*,*,#6191,.F.);
#8353=ORIENTED_EDGE('',*,*,#6202,.T.);
#8354=ORIENTED_EDGE('',*,*,#6105,.T.);
#8355=ORIENTED_EDGE('',*,*,#6193,.F.);
#8356=ORIENTED_EDGE('',*,*,#6069,.T.);
#8357=ORIENTED_EDGE('',*,*,#6203,.T.);
#8358=ORIENTED_EDGE('',*,*,#6197,.F.);
#8359=ORIENTED_EDGE('',*,*,#6107,.T.);
#8360=ORIENTED_EDGE('',*,*,#6204,.T.);
#8361=ORIENTED_EDGE('',*,*,#6201,.F.);
#8362=ORIENTED_EDGE('',*,*,#6190,.F.);
#8363=ORIENTED_EDGE('',*,*,#6083,.F.);
#8364=ORIENTED_EDGE('',*,*,#6046,.T.);
#8365=ORIENTED_EDGE('',*,*,#6205,.T.);
#8366=ORIENTED_EDGE('',*,*,#6206,.T.);
#8367=ORIENTED_EDGE('',*,*,#6200,.F.);
#8368=ORIENTED_EDGE('',*,*,#6198,.F.);
#8369=ORIENTED_EDGE('',*,*,#6204,.F.);
#8370=ORIENTED_EDGE('',*,*,#6207,.T.);
#8371=ORIENTED_EDGE('',*,*,#6208,.F.);
#8372=ORIENTED_EDGE('',*,*,#6044,.T.);
#8373=ORIENTED_EDGE('',*,*,#5966,.F.);
#8374=ORIENTED_EDGE('',*,*,#6001,.F.);
#8375=ORIENTED_EDGE('',*,*,#5992,.F.);
#8376=ORIENTED_EDGE('',*,*,#5968,.F.);
#8377=ORIENTED_EDGE('',*,*,#6166,.T.);
#8378=ORIENTED_EDGE('',*,*,#6121,.F.);
#8379=ORIENTED_EDGE('',*,*,#5897,.T.);
#8380=ORIENTED_EDGE('',*,*,#6209,.T.);
#8381=ORIENTED_EDGE('',*,*,#6210,.T.);
#8382=ORIENTED_EDGE('',*,*,#6202,.F.);
#8383=ORIENTED_EDGE('',*,*,#6192,.F.);
#8384=ORIENTED_EDGE('',*,*,#6211,.T.);
#8385=ORIENTED_EDGE('',*,*,#6212,.T.);
#8386=ORIENTED_EDGE('',*,*,#6209,.F.);
#8387=ORIENTED_EDGE('',*,*,#5896,.T.);
#8388=ORIENTED_EDGE('',*,*,#6203,.F.);
#8389=ORIENTED_EDGE('',*,*,#6213,.T.);
#8390=ORIENTED_EDGE('',*,*,#6211,.F.);
#8391=ORIENTED_EDGE('',*,*,#5895,.T.);
#8392=ORIENTED_EDGE('',*,*,#6196,.F.);
#8393=ORIENTED_EDGE('',*,*,#6194,.F.);
#8394=ORIENTED_EDGE('',*,*,#6208,.T.);
#8395=ORIENTED_EDGE('',*,*,#6214,.T.);
#8396=ORIENTED_EDGE('',*,*,#6205,.F.);
#8397=ORIENTED_EDGE('',*,*,#6045,.T.);
#8398=ORIENTED_EDGE('',*,*,#6210,.F.);
#8399=ORIENTED_EDGE('',*,*,#6215,.T.);
#8400=ORIENTED_EDGE('',*,*,#6207,.F.);
#8401=ORIENTED_EDGE('',*,*,#6106,.T.);
#8402=ORIENTED_EDGE('',*,*,#6212,.F.);
#8403=ORIENTED_EDGE('',*,*,#6216,.F.);
#8404=ORIENTED_EDGE('',*,*,#6214,.F.);
#8405=ORIENTED_EDGE('',*,*,#6215,.F.);
#8406=ORIENTED_EDGE('',*,*,#6154,.T.);
#8407=ORIENTED_EDGE('',*,*,#6213,.F.);
#8408=ORIENTED_EDGE('',*,*,#6068,.T.);
#8409=ORIENTED_EDGE('',*,*,#6206,.F.);
#8410=ORIENTED_EDGE('',*,*,#6216,.T.);
#11483=PLANE('',#12615);
#11484=PLANE('',#12616);
#11485=PLANE('',#12620);
#11486=PLANE('',#12621);
#11487=PLANE('',#12622);
#11488=PLANE('',#12623);
#11489=PLANE('',#12624);
#11490=PLANE('',#12625);
#11491=PLANE('',#12626);
#11492=PLANE('',#12627);
#11493=PLANE('',#12628);
#11494=PLANE('',#12629);
#11495=PLANE('',#12630);
#11496=PLANE('',#12632);
#11497=PLANE('',#12633);
#11498=PLANE('',#12634);
#11499=PLANE('',#12635);
#11500=PLANE('',#12636);
#11501=PLANE('',#12637);
#11502=PLANE('',#12638);
#11503=PLANE('',#12639);
#11504=PLANE('',#12640);
#11505=PLANE('',#12641);
#11506=PLANE('',#12642);
#11507=PLANE('',#12643);
#11508=PLANE('',#12645);
#11509=PLANE('',#12646);
#11510=PLANE('',#12647);
#11511=PLANE('',#12648);
#11512=PLANE('',#12649);
#11513=PLANE('',#12650);
#11514=PLANE('',#12651);
#11515=PLANE('',#12652);
#11516=PLANE('',#12653);
#11517=PLANE('',#12654);
#11518=PLANE('',#12655);
#11519=PLANE('',#12656);
#11520=PLANE('',#12657);
#11521=PLANE('',#12658);
#11522=PLANE('',#12659);
#11523=PLANE('',#12663);
#11524=PLANE('',#12664);
#11525=PLANE('',#12665);
#11526=PLANE('',#12666);
#11527=PLANE('',#12667);
#11528=PLANE('',#12672);
#11529=PLANE('',#12673);
#11530=PLANE('',#12674);
#11531=PLANE('',#12675);
#11532=PLANE('',#12676);
#11533=PLANE('',#12677);
#11534=PLANE('',#12678);
#11535=PLANE('',#12679);
#11536=PLANE('',#12684);
#11537=PLANE('',#12685);
#11538=PLANE('',#12686);
#11539=PLANE('',#12687);
#11540=PLANE('',#12688);
#11541=PLANE('',#12689);
#11542=PLANE('',#12715);
#11543=PLANE('',#12719);
#11544=PLANE('',#12729);
#11545=PLANE('',#12733);
#11546=PLANE('',#12742);
#11547=PLANE('',#12746);
#11548=PLANE('',#12751);
#11549=PLANE('',#12752);
#11550=PLANE('',#12753);
#11551=PLANE('',#12754);
#11552=PLANE('',#12755);
#11553=PLANE('',#12756);
#11554=PLANE('',#12757);
#11555=PLANE('',#12764);
#11556=PLANE('',#12774);
#11786=ADVANCED_FACE('',(#1819),#11483,.T.);
#11787=ADVANCED_FACE('',(#1820,#1340),#11484,.T.);
#11788=ADVANCED_FACE('',(#1821),#11485,.T.);
#11789=ADVANCED_FACE('',(#1822),#11486,.T.);
#11790=ADVANCED_FACE('',(#1823),#11487,.T.);
#11791=ADVANCED_FACE('',(#1824),#11488,.T.);
#11792=ADVANCED_FACE('',(#1825),#11489,.T.);
#11793=ADVANCED_FACE('',(#1826),#11490,.T.);
#11794=ADVANCED_FACE('',(#1827),#11491,.T.);
#11795=ADVANCED_FACE('',(#1828),#11492,.T.);
#11796=ADVANCED_FACE('',(#1829),#11493,.T.);
#11797=ADVANCED_FACE('',(#1830),#11494,.T.);
#11798=ADVANCED_FACE('',(#1831,#1341),#11495,.T.);
#11799=ADVANCED_FACE('',(#1832),#11496,.T.);
#11800=ADVANCED_FACE('',(#1833),#11497,.T.);
#11801=ADVANCED_FACE('',(#1834),#11498,.T.);
#11802=ADVANCED_FACE('',(#1835),#11499,.T.);
#11803=ADVANCED_FACE('',(#1836),#11500,.T.);
#11804=ADVANCED_FACE('',(#1837),#11501,.T.);
#11805=ADVANCED_FACE('',(#1838),#11502,.T.);
#11806=ADVANCED_FACE('',(#1839),#11503,.T.);
#11807=ADVANCED_FACE('',(#1840),#11504,.T.);
#11808=ADVANCED_FACE('',(#1841),#11505,.T.);
#11809=ADVANCED_FACE('',(#1842),#11506,.T.);
#11810=ADVANCED_FACE('',(#1843,#1342),#11507,.T.);
#11811=ADVANCED_FACE('',(#1844),#11508,.T.);
#11812=ADVANCED_FACE('',(#1845),#11509,.T.);
#11813=ADVANCED_FACE('',(#1846),#11510,.T.);
#11814=ADVANCED_FACE('',(#1847),#11511,.T.);
#11815=ADVANCED_FACE('',(#1848),#11512,.T.);
#11816=ADVANCED_FACE('',(#1849),#11513,.T.);
#11817=ADVANCED_FACE('',(#1850),#11514,.T.);
#11818=ADVANCED_FACE('',(#1851),#11515,.T.);
#11819=ADVANCED_FACE('',(#1852),#11516,.T.);
#11820=ADVANCED_FACE('',(#1853),#11517,.T.);
#11821=ADVANCED_FACE('',(#1854),#11518,.T.);
#11822=ADVANCED_FACE('',(#1855),#11519,.T.);
#11823=ADVANCED_FACE('',(#1856),#11520,.T.);
#11824=ADVANCED_FACE('',(#1857),#11521,.T.);
#11825=ADVANCED_FACE('',(#1858,#1343),#11522,.T.);
#11826=ADVANCED_FACE('',(#1859),#11523,.T.);
#11827=ADVANCED_FACE('',(#1860),#11524,.T.);
#11828=ADVANCED_FACE('',(#1861),#11525,.T.);
#11829=ADVANCED_FACE('',(#1862),#11526,.T.);
#11830=ADVANCED_FACE('',(#1863),#1186,.T.);
#11831=ADVANCED_FACE('',(#1864),#1187,.F.);
#11832=ADVANCED_FACE('',(#1865,#1344,#1345,#1346,#1347),#11527,.T.);
#11833=ADVANCED_FACE('',(#1866),#1188,.T.);
#11834=ADVANCED_FACE('',(#1867),#11528,.T.);
#11835=ADVANCED_FACE('',(#1868),#11529,.T.);
#11836=ADVANCED_FACE('',(#1869),#11530,.T.);
#11837=ADVANCED_FACE('',(#1870),#11531,.T.);
#11838=ADVANCED_FACE('',(#1871),#11532,.T.);
#11839=ADVANCED_FACE('',(#1872),#1189,.T.);
#11840=ADVANCED_FACE('',(#1873),#1190,.F.);
#11841=ADVANCED_FACE('',(#1874),#11533,.T.);
#11842=ADVANCED_FACE('',(#1875),#11534,.T.);
#11843=ADVANCED_FACE('',(#1876),#1191,.T.);
#11844=ADVANCED_FACE('',(#1877),#1192,.F.);
#11845=ADVANCED_FACE('',(#1878,#1348,#1349,#1350,#1351),#11535,.T.);
#11846=ADVANCED_FACE('',(#1879),#1193,.T.);
#11847=ADVANCED_FACE('',(#1880),#11536,.T.);
#11848=ADVANCED_FACE('',(#1881),#11537,.T.);
#11849=ADVANCED_FACE('',(#1882),#11538,.T.);
#11850=ADVANCED_FACE('',(#1883),#11539,.T.);
#11851=ADVANCED_FACE('',(#1884),#11540,.T.);
#11852=ADVANCED_FACE('',(#1885),#11541,.T.);
#11853=ADVANCED_FACE('',(#1886),#1194,.T.);
#11854=ADVANCED_FACE('',(#1887),#1195,.F.);
#11855=ADVANCED_FACE('',(#1888),#362,.F.);
#11856=ADVANCED_FACE('',(#1889),#246,.F.);
#11857=ADVANCED_FACE('',(#1890),#363,.F.);
#11858=ADVANCED_FACE('',(#1891),#364,.F.);
#11859=ADVANCED_FACE('',(#1892),#247,.F.);
#11860=ADVANCED_FACE('',(#1893),#365,.F.);
#11861=ADVANCED_FACE('',(#1894),#366,.F.);
#11862=ADVANCED_FACE('',(#1895),#248,.F.);
#11863=ADVANCED_FACE('',(#1896),#367,.F.);
#11864=ADVANCED_FACE('',(#1897),#368,.F.);
#11865=ADVANCED_FACE('',(#1898),#249,.F.);
#11866=ADVANCED_FACE('',(#1899),#369,.F.);
#11867=ADVANCED_FACE('',(#1900),#370,.F.);
#11868=ADVANCED_FACE('',(#1901),#250,.F.);
#11869=ADVANCED_FACE('',(#1902,#1352),#11542,.F.);
#11870=ADVANCED_FACE('',(#1903),#251,.F.);
#11871=ADVANCED_FACE('',(#1904,#1353),#11543,.F.);
#11872=ADVANCED_FACE('',(#1905),#252,.F.);
#11873=ADVANCED_FACE('',(#1906),#371,.F.);
#11874=ADVANCED_FACE('',(#1907),#372,.F.);
#11875=ADVANCED_FACE('',(#1908),#253,.F.);
#11876=ADVANCED_FACE('',(#1909,#1354),#11544,.F.);
#11877=ADVANCED_FACE('',(#1910),#254,.F.);
#11878=ADVANCED_FACE('',(#1911,#1355),#11545,.F.);
#11879=ADVANCED_FACE('',(#1912),#255,.F.);
#11880=ADVANCED_FACE('',(#1913),#373,.F.);
#11881=ADVANCED_FACE('',(#1914),#374,.F.);
#11882=ADVANCED_FACE('',(#1915),#256,.F.);
#11883=ADVANCED_FACE('',(#1916,#1356),#11546,.F.);
#11884=ADVANCED_FACE('',(#1917),#257,.F.);
#11885=ADVANCED_FACE('',(#1918,#1357),#11547,.F.);
#11886=ADVANCED_FACE('',(#1919),#258,.F.);
#11887=ADVANCED_FACE('',(#1920),#375,.F.);
#11888=ADVANCED_FACE('',(#1921),#1196,.T.);
#11889=ADVANCED_FACE('',(#1922),#1197,.T.);
#11890=ADVANCED_FACE('',(#1923),#11548,.T.);
#11891=ADVANCED_FACE('',(#1924),#11549,.T.);
#11892=ADVANCED_FACE('',(#1925),#11550,.T.);
#11893=ADVANCED_FACE('',(#1926),#11551,.T.);
#11894=ADVANCED_FACE('',(#1927),#11552,.T.);
#11895=ADVANCED_FACE('',(#1928),#11553,.T.);
#11896=ADVANCED_FACE('',(#1929),#11554,.T.);
#11897=ADVANCED_FACE('',(#1930),#1198,.T.);
#11898=ADVANCED_FACE('',(#1931),#1199,.T.);
#11899=ADVANCED_FACE('',(#1932),#1200,.T.);
#11900=ADVANCED_FACE('',(#1933),#1201,.T.);
#11901=ADVANCED_FACE('',(#1934),#1202,.F.);
#11902=ADVANCED_FACE('',(#1935),#1203,.F.);
#11903=ADVANCED_FACE('',(#1936),#1204,.F.);
#11904=ADVANCED_FACE('',(#1937),#1205,.F.);
#11905=ADVANCED_FACE('',(#1938),#227,.F.);
#11906=ADVANCED_FACE('',(#1939),#228,.F.);
#11907=ADVANCED_FACE('',(#1940,#1358),#11555,.T.);
#11908=ADVANCED_FACE('',(#1941),#229,.F.);
#11909=ADVANCED_FACE('',(#1942),#259,.F.);
#11910=ADVANCED_FACE('',(#1943),#230,.F.);
#11911=ADVANCED_FACE('',(#1944),#260,.F.);
#11912=ADVANCED_FACE('',(#1945),#261,.T.);
#11913=ADVANCED_FACE('',(#1946,#1359),#11556,.T.);
#11914=ADVANCED_FACE('',(#1947),#262,.T.);
#12480=CLOSED_SHELL('',(#11786,#11787,#11788,#11789,#11790,#11791,#11792,
#11793,#11794,#11795,#11796,#11797,#11798,#11799,#11800,#11801,#11802,#11803,
#11804,#11805,#11806,#11807,#11808,#11809,#11810,#11811,#11812,#11813,#11814,
#11815,#11816,#11817,#11818,#11819,#11820,#11821,#11822,#11823,#11824,#11825,
#11826,#11827,#11828,#11829,#11830,#11831,#11832,#11833,#11834,#11835,#11836,
#11837,#11838,#11839,#11840,#11841,#11842,#11843,#11844,#11845,#11846,#11847,
#11848,#11849,#11850,#11851,#11852,#11853,#11854,#11855,#11856,#11857,#11858,
#11859,#11860,#11861,#11862,#11863,#11864,#11865,#11866,#11867,#11868,#11869,
#11870,#11871,#11872,#11873,#11874,#11875,#11876,#11877,#11878,#11879,#11880,
#11881,#11882,#11883,#11884,#11885,#11886,#11887,#11888,#11889,#11890,#11891,
#11892,#11893,#11894,#11895,#11896,#11897,#11898,#11899,#11900,#11901,#11902,
#11903,#11904,#11905,#11906,#11907,#11908,#11909,#11910,#11911,#11912,#11913,
#11914));
#12614=AXIS2_PLACEMENT_3D('',#16340,#13622,#13623);
#12615=AXIS2_PLACEMENT_3D('',#16341,#13624,#13625);
#12616=AXIS2_PLACEMENT_3D('',#16354,#13632,#13633);
#12617=AXIS2_PLACEMENT_3D('',#16358,#13635,#13636);
#12618=AXIS2_PLACEMENT_3D('',#16362,#13638,#13639);
#12619=AXIS2_PLACEMENT_3D('',#16365,#13641,#13642);
#12620=AXIS2_PLACEMENT_3D('',#16366,#13643,#13644);
#12621=AXIS2_PLACEMENT_3D('',#16372,#13648,#13649);
#12622=AXIS2_PLACEMENT_3D('',#16382,#13655,#13656);
#12623=AXIS2_PLACEMENT_3D('',#16392,#13662,#13663);
#12624=AXIS2_PLACEMENT_3D('',#16398,#13667,#13668);
#12625=AXIS2_PLACEMENT_3D('',#16406,#13673,#13674);
#12626=AXIS2_PLACEMENT_3D('',#16413,#13679,#13680);
#12627=AXIS2_PLACEMENT_3D('',#16421,#13685,#13686);
#12628=AXIS2_PLACEMENT_3D('',#16425,#13689,#13690);
#12629=AXIS2_PLACEMENT_3D('',#16435,#13696,#13697);
#12630=AXIS2_PLACEMENT_3D('',#16445,#13703,#13704);
#12631=AXIS2_PLACEMENT_3D('',#16452,#13708,#13709);
#12632=AXIS2_PLACEMENT_3D('',#16453,#13710,#13711);
#12633=AXIS2_PLACEMENT_3D('',#16461,#13716,#13717);
#12634=AXIS2_PLACEMENT_3D('',#16466,#13721,#13722);
#12635=AXIS2_PLACEMENT_3D('',#16474,#13727,#13728);
#12636=AXIS2_PLACEMENT_3D('',#16478,#13731,#13732);
#12637=AXIS2_PLACEMENT_3D('',#16488,#13738,#13739);
#12638=AXIS2_PLACEMENT_3D('',#16492,#13742,#13743);
#12639=AXIS2_PLACEMENT_3D('',#16500,#13748,#13749);
#12640=AXIS2_PLACEMENT_3D('',#16508,#13754,#13755);
#12641=AXIS2_PLACEMENT_3D('',#16521,#13762,#13763);
#12642=AXIS2_PLACEMENT_3D('',#16530,#13769,#13770);
#12643=AXIS2_PLACEMENT_3D('',#16538,#13775,#13776);
#12644=AXIS2_PLACEMENT_3D('',#16543,#13779,#13780);
#12645=AXIS2_PLACEMENT_3D('',#16544,#13781,#13782);
#12646=AXIS2_PLACEMENT_3D('',#16552,#13787,#13788);
#12647=AXIS2_PLACEMENT_3D('',#16554,#13790,#13791);
#12648=AXIS2_PLACEMENT_3D('',#16562,#13796,#13797);
#12649=AXIS2_PLACEMENT_3D('',#16567,#13801,#13802);
#12650=AXIS2_PLACEMENT_3D('',#16575,#13807,#13808);
#12651=AXIS2_PLACEMENT_3D('',#16585,#13814,#13815);
#12652=AXIS2_PLACEMENT_3D('',#16595,#13821,#13822);
#12653=AXIS2_PLACEMENT_3D('',#16601,#13826,#13827);
#12654=AXIS2_PLACEMENT_3D('',#16609,#13832,#13833);
#12655=AXIS2_PLACEMENT_3D('',#16616,#13838,#13839);
#12656=AXIS2_PLACEMENT_3D('',#16624,#13844,#13845);
#12657=AXIS2_PLACEMENT_3D('',#16628,#13848,#13849);
#12658=AXIS2_PLACEMENT_3D('',#16638,#13855,#13856);
#12659=AXIS2_PLACEMENT_3D('',#16648,#13862,#13863);
#12660=AXIS2_PLACEMENT_3D('',#16652,#13865,#13866);
#12661=AXIS2_PLACEMENT_3D('',#16656,#13868,#13869);
#12662=AXIS2_PLACEMENT_3D('',#16659,#13871,#13872);
#12663=AXIS2_PLACEMENT_3D('',#16660,#13873,#13874);
#12664=AXIS2_PLACEMENT_3D('',#16666,#13878,#13879);
#12665=AXIS2_PLACEMENT_3D('',#16671,#13883,#13884);
#12666=AXIS2_PLACEMENT_3D('',#16677,#13888,#13889);
#12667=AXIS2_PLACEMENT_3D('',#16738,#13893,#13894);
#12668=AXIS2_PLACEMENT_3D('',#16791,#13901,#13902);
#12669=AXIS2_PLACEMENT_3D('',#16793,#13903,#13904);
#12670=AXIS2_PLACEMENT_3D('',#16795,#13905,#13906);
#12671=AXIS2_PLACEMENT_3D('',#16797,#13907,#13908);
#12672=AXIS2_PLACEMENT_3D('',#16821,#13911,#13912);
#12673=AXIS2_PLACEMENT_3D('',#16824,#13915,#13916);
#12674=AXIS2_PLACEMENT_3D('',#16825,#13917,#13918);
#12675=AXIS2_PLACEMENT_3D('',#16828,#13921,#13922);
#12676=AXIS2_PLACEMENT_3D('',#16829,#13923,#13924);
#12677=AXIS2_PLACEMENT_3D('',#16876,#13926,#13927);
#12678=AXIS2_PLACEMENT_3D('',#16882,#13931,#13932);
#12679=AXIS2_PLACEMENT_3D('',#16943,#13936,#13937);
#12680=AXIS2_PLACEMENT_3D('',#16995,#13944,#13945);
#12681=AXIS2_PLACEMENT_3D('',#16997,#13946,#13947);
#12682=AXIS2_PLACEMENT_3D('',#16999,#13948,#13949);
#12683=AXIS2_PLACEMENT_3D('',#17001,#13950,#13951);
#12684=AXIS2_PLACEMENT_3D('',#17025,#13954,#13955);
#12685=AXIS2_PLACEMENT_3D('',#17030,#13959,#13960);
#12686=AXIS2_PLACEMENT_3D('',#17032,#13962,#13963);
#12687=AXIS2_PLACEMENT_3D('',#17033,#13964,#13965);
#12688=AXIS2_PLACEMENT_3D('',#17036,#13968,#13969);
#12689=AXIS2_PLACEMENT_3D('',#17038,#13971,#13972);
#12690=AXIS2_PLACEMENT_3D('',#17085,#13974,#13975);
#12691=AXIS2_PLACEMENT_3D('',#17088,#13977,#13978);
#12692=AXIS2_PLACEMENT_3D('',#17089,#13979,#13980);
#12693=AXIS2_PLACEMENT_3D('',#17091,#13981,#13982);
#12694=AXIS2_PLACEMENT_3D('',#17093,#13984,#13985);
#12695=AXIS2_PLACEMENT_3D('',#17095,#13987,#13988);
#12696=AXIS2_PLACEMENT_3D('',#17098,#13990,#13991);
#12697=AXIS2_PLACEMENT_3D('',#17099,#13992,#13993);
#12698=AXIS2_PLACEMENT_3D('',#17101,#13994,#13995);
#12699=AXIS2_PLACEMENT_3D('',#17103,#13997,#13998);
#12700=AXIS2_PLACEMENT_3D('',#17105,#14000,#14001);
#12701=AXIS2_PLACEMENT_3D('',#17108,#14003,#14004);
#12702=AXIS2_PLACEMENT_3D('',#17109,#14005,#14006);
#12703=AXIS2_PLACEMENT_3D('',#17111,#14007,#14008);
#12704=AXIS2_PLACEMENT_3D('',#17113,#14010,#14011);
#12705=AXIS2_PLACEMENT_3D('',#17115,#14013,#14014);
#12706=AXIS2_PLACEMENT_3D('',#17118,#14016,#14017);
#12707=AXIS2_PLACEMENT_3D('',#17119,#14018,#14019);
#12708=AXIS2_PLACEMENT_3D('',#17121,#14020,#14021);
#12709=AXIS2_PLACEMENT_3D('',#17123,#14023,#14024);
#12710=AXIS2_PLACEMENT_3D('',#17125,#14026,#14027);
#12711=AXIS2_PLACEMENT_3D('',#17127,#14028,#14029);
#12712=AXIS2_PLACEMENT_3D('',#17130,#14031,#14032);
#12713=AXIS2_PLACEMENT_3D('',#17131,#14033,#14034);
#12714=AXIS2_PLACEMENT_3D('',#17134,#14036,#14037);
#12715=AXIS2_PLACEMENT_3D('',#17135,#14038,#14039);
#12716=AXIS2_PLACEMENT_3D('',#17137,#14040,#14041);
#12717=AXIS2_PLACEMENT_3D('',#17138,#14042,#14043);
#12718=AXIS2_PLACEMENT_3D('',#17141,#14045,#14046);
#12719=AXIS2_PLACEMENT_3D('',#17142,#14047,#14048);
#12720=AXIS2_PLACEMENT_3D('',#17144,#14049,#14050);
#12721=AXIS2_PLACEMENT_3D('',#17145,#14051,#14052);
#12722=AXIS2_PLACEMENT_3D('',#17148,#14054,#14055);
#12723=AXIS2_PLACEMENT_3D('',#17149,#14056,#14057);
#12724=AXIS2_PLACEMENT_3D('',#17152,#14059,#14060);
#12725=AXIS2_PLACEMENT_3D('',#17153,#14061,#14062);
#12726=AXIS2_PLACEMENT_3D('',#17156,#14064,#14065);
#12727=AXIS2_PLACEMENT_3D('',#17157,#14066,#14067);
#12728=AXIS2_PLACEMENT_3D('',#17160,#14069,#14070);
#12729=AXIS2_PLACEMENT_3D('',#17161,#14071,#14072);
#12730=AXIS2_PLACEMENT_3D('',#17163,#14073,#14074);
#12731=AXIS2_PLACEMENT_3D('',#17164,#14075,#14076);
#12732=AXIS2_PLACEMENT_3D('',#17167,#14078,#14079);
#12733=AXIS2_PLACEMENT_3D('',#17168,#14080,#14081);
#12734=AXIS2_PLACEMENT_3D('',#17170,#14082,#14083);
#12735=AXIS2_PLACEMENT_3D('',#17171,#14084,#14085);
#12736=AXIS2_PLACEMENT_3D('',#17174,#14087,#14088);
#12737=AXIS2_PLACEMENT_3D('',#17175,#14089,#14090);
#12738=AXIS2_PLACEMENT_3D('',#17177,#14092,#14093);
#12739=AXIS2_PLACEMENT_3D('',#17180,#14095,#14096);
#12740=AXIS2_PLACEMENT_3D('',#17181,#14097,#14098);
#12741=AXIS2_PLACEMENT_3D('',#17184,#14100,#14101);
#12742=AXIS2_PLACEMENT_3D('',#17185,#14102,#14103);
#12743=AXIS2_PLACEMENT_3D('',#17187,#14104,#14105);
#12744=AXIS2_PLACEMENT_3D('',#17188,#14106,#14107);
#12745=AXIS2_PLACEMENT_3D('',#17191,#14109,#14110);
#12746=AXIS2_PLACEMENT_3D('',#17192,#14111,#14112);
#12747=AXIS2_PLACEMENT_3D('',#17194,#14113,#14114);
#12748=AXIS2_PLACEMENT_3D('',#17195,#14115,#14116);
#12749=AXIS2_PLACEMENT_3D('',#17198,#14118,#14119);
#12750=AXIS2_PLACEMENT_3D('',#17199,#14120,#14121);
#12751=AXIS2_PLACEMENT_3D('',#17296,#14123,#14124);
#12752=AXIS2_PLACEMENT_3D('',#17297,#14125,#14126);
#12753=AXIS2_PLACEMENT_3D('',#17298,#14127,#14128);
#12754=AXIS2_PLACEMENT_3D('',#17299,#14129,#14130);
#12755=AXIS2_PLACEMENT_3D('',#17300,#14131,#14132);
#12756=AXIS2_PLACEMENT_3D('',#17301,#14133,#14134);
#12757=AXIS2_PLACEMENT_3D('',#17302,#14135,#14136);
#12758=AXIS2_PLACEMENT_3D('',#17527,#14139,#14140);
#12759=AXIS2_PLACEMENT_3D('',#17529,#14141,#14142);
#12760=AXIS2_PLACEMENT_3D('',#17530,#14143,#14144);
#12761=AXIS2_PLACEMENT_3D('',#17531,#14145,#14146);
#12762=AXIS2_PLACEMENT_3D('',#17533,#14147,#14148);
#12763=AXIS2_PLACEMENT_3D('',#17534,#14149,#14150);
#12764=AXIS2_PLACEMENT_3D('',#17535,#14151,#14152);
#12765=AXIS2_PLACEMENT_3D('',#17536,#14153,#14154);
#12766=AXIS2_PLACEMENT_3D('',#17538,#14155,#14156);
#12767=AXIS2_PLACEMENT_3D('',#17539,#14157,#14158);
#12768=AXIS2_PLACEMENT_3D('',#17540,#14159,#14160);
#12769=AXIS2_PLACEMENT_3D('',#17542,#14161,#14162);
#12770=AXIS2_PLACEMENT_3D('',#17544,#14164,#14165);
#12771=AXIS2_PLACEMENT_3D('',#17545,#14166,#14167);
#12772=AXIS2_PLACEMENT_3D('',#17546,#14168,#14169);
#12773=AXIS2_PLACEMENT_3D('',#17548,#14171,#14172);
#12774=AXIS2_PLACEMENT_3D('',#17550,#14174,#14175);
#12775=AXIS2_PLACEMENT_3D('',#17552,#14177,#14178);
#13622=DIRECTION('axis',(0.,0.,1.));
#13623=DIRECTION('refdir',(1.,0.,0.));
#13624=DIRECTION('center_axis',(-0.923879532511287,0.,-0.382683432365089));
#13625=DIRECTION('ref_axis',(-0.382683432365089,0.,0.923879532511287));
#13626=DIRECTION('',(0.336556770590777,-0.475963149477969,-0.812519920068745));
#13627=DIRECTION('',(0.,-1.,0.));
#13628=DIRECTION('',(-0.336556770590777,-0.475963149477969,0.812519920068745));
#13629=DIRECTION('',(-0.357406744336593,0.357406744336593,0.862856209461017));
#13630=DIRECTION('',(0.,1.,0.));
#13631=DIRECTION('',(0.357406744336593,0.357406744336593,-0.862856209461017));
#13632=DIRECTION('center_axis',(-1.,0.,0.));
#13633=DIRECTION('ref_axis',(0.,0.,1.));
#13634=DIRECTION('',(0.,0.,-1.));
#13635=DIRECTION('center_axis',(-1.,0.,0.));
#13636=DIRECTION('ref_axis',(0.,-0.707106781186547,-0.707106781186548));
#13637=DIRECTION('',(0.,-1.,0.));
#13638=DIRECTION('center_axis',(-1.,0.,0.));
#13639=DIRECTION('ref_axis',(0.,0.707106781186547,-0.707106781186548));
#13640=DIRECTION('',(0.,0.,1.));
#13641=DIRECTION('center_axis',(1.,0.,0.));
#13642=DIRECTION('ref_axis',(0.,0.,1.));
#13643=DIRECTION('center_axis',(-0.707106781186548,-0.707106781186548,0.));
#13644=DIRECTION('ref_axis',(0.,0.,1.));
#13645=DIRECTION('',(0.707106781186548,-0.707106781186548,0.));
#13646=DIRECTION('',(0.,0.,-1.));
#13647=DIRECTION('',(-0.707106781186548,0.707106781186548,0.));
#13648=DIRECTION('center_axis',(-0.577350269189626,-0.577350269189626,-0.577350269189626));
#13649=DIRECTION('ref_axis',(-0.707106781186548,0.,0.707106781186547));
#13650=DIRECTION('',(-0.707106781186548,0.,0.707106781186547));
#13651=DIRECTION('',(-0.812519920068745,0.475963149477971,0.336556770590774));
#13652=DIRECTION('',(0.,0.707106781186548,-0.707106781186548));
#13653=DIRECTION('',(0.475963149477967,0.336556770590778,-0.812519920068745));
#13654=DIRECTION('',(0.812519920068746,-0.336556770590778,-0.475963149477967));
#13655=DIRECTION('center_axis',(-0.382683432365086,0.,-0.923879532511288));
#13656=DIRECTION('ref_axis',(-0.923879532511288,0.,0.382683432365086));
#13657=DIRECTION('',(0.,1.,0.));
#13658=DIRECTION('',(0.812519920068745,0.475963149477971,-0.336556770590774));
#13659=DIRECTION('',(0.862856209461019,-0.35740674433659,-0.35740674433659));
#13660=DIRECTION('',(0.,-1.,0.));
#13661=DIRECTION('',(-0.862856209461019,-0.35740674433659,0.35740674433659));
#13662=DIRECTION('center_axis',(0.,0.,-1.));
#13663=DIRECTION('ref_axis',(-1.,0.,0.));
#13664=DIRECTION('',(-1.,0.,0.));
#13665=DIRECTION('',(0.,1.,0.));
#13666=DIRECTION('',(1.,0.,0.));
#13667=DIRECTION('center_axis',(0.,0.707106781186548,-0.707106781186548));
#13668=DIRECTION('ref_axis',(-1.,0.,0.));
#13669=DIRECTION('',(0.,0.707106781186548,0.707106781186548));
#13670=DIRECTION('',(-1.,0.,0.));
#13671=DIRECTION('',(0.,-0.707106781186548,-0.707106781186548));
#13672=DIRECTION('',(0.862856209461016,0.357406744336594,0.357406744336594));
#13673=DIRECTION('center_axis',(-0.577350269189626,0.577350269189626,-0.577350269189626));
#13674=DIRECTION('ref_axis',(-0.707106781186548,0.,0.707106781186547));
#13675=DIRECTION('',(-0.707106781186548,-0.707106781186548,0.));
#13676=DIRECTION('',(-0.812519920068746,-0.336556770590778,0.475963149477967));
#13677=DIRECTION('',(-0.475963149477968,0.336556770590778,0.812519920068745));
#13678=DIRECTION('',(0.707106781186548,0.,-0.707106781186547));
#13679=DIRECTION('center_axis',(0.38268343236509,0.,-0.923879532511287));
#13680=DIRECTION('ref_axis',(-0.923879532511287,0.,-0.38268343236509));
#13681=DIRECTION('',(0.812519920068746,-0.475963149477968,0.336556770590778));
#13682=DIRECTION('',(0.,-1.,0.));
#13683=DIRECTION('',(-0.812519920068746,-0.475963149477968,-0.336556770590778));
#13684=DIRECTION('',(-0.862856209461016,0.357406744336594,-0.357406744336594));
#13685=DIRECTION('center_axis',(0.,-0.707106781186548,-0.707106781186548));
#13686=DIRECTION('ref_axis',(-1.,0.,0.));
#13687=DIRECTION('',(0.,-0.707106781186548,0.707106781186548));
#13688=DIRECTION('',(1.,0.,0.));
#13689=DIRECTION('center_axis',(0.577350269189626,-0.577350269189626,-0.577350269189626));
#13690=DIRECTION('ref_axis',(-0.707106781186548,0.,-0.707106781186548));
#13691=DIRECTION('',(-0.707106781186548,0.,-0.707106781186548));
#13692=DIRECTION('',(-0.336556770590791,0.475963149477956,-0.812519920068747));
#13693=DIRECTION('',(0.707106781186548,0.707106781186548,0.));
#13694=DIRECTION('',(0.812519920068746,0.336556770590782,0.475963149477964));
#13695=DIRECTION('',(0.475963149477967,-0.336556770590778,0.812519920068745));
#13696=DIRECTION('center_axis',(0.923879532511282,0.,-0.382683432365102));
#13697=DIRECTION('ref_axis',(-0.382683432365102,0.,-0.923879532511282));
#13698=DIRECTION('',(0.,1.,0.));
#13699=DIRECTION('',(0.336556770590791,0.475963149477956,0.812519920068747));
#13700=DIRECTION('',(0.357406744336604,-0.357406744336604,0.862856209461008));
#13701=DIRECTION('',(0.,-1.,0.));
#13702=DIRECTION('',(-0.357406744336604,-0.357406744336604,-0.862856209461008));
#13703=DIRECTION('center_axis',(1.,0.,0.));
#13704=DIRECTION('ref_axis',(0.,0.,-1.));
#13705=DIRECTION('',(0.,0.,-1.));
#13706=DIRECTION('',(0.,1.,0.));
#13707=DIRECTION('',(0.,0.,1.));
#13708=DIRECTION('center_axis',(-1.,0.,0.));
#13709=DIRECTION('ref_axis',(0.,0.,1.));
#13710=DIRECTION('center_axis',(0.707106781186548,0.707106781186548,0.));
#13711=DIRECTION('ref_axis',(0.,0.,-1.));
#13712=DIRECTION('',(-0.707106781186548,0.707106781186548,0.));
#13713=DIRECTION('',(0.,0.,-1.));
#13714=DIRECTION('',(0.707106781186548,-0.707106781186548,1.57009245868377E-14));
#13715=DIRECTION('',(-0.357406744336597,0.357406744336597,0.862856209461013));
#13716=DIRECTION('center_axis',(0.577350269189626,0.577350269189626,-0.577350269189626));
#13717=DIRECTION('ref_axis',(-0.707106781186548,0.,-0.707106781186548));
#13718=DIRECTION('',(-0.475963149477967,-0.336556770590778,-0.812519920068745));
#13719=DIRECTION('',(-0.812519920068746,0.336556770590782,-0.475963149477964));
#13720=DIRECTION('',(0.707106781186548,0.,0.707106781186548));
#13721=DIRECTION('center_axis',(0.923879532511285,0.,0.382683432365095));
#13722=DIRECTION('ref_axis',(0.382683432365095,0.,-0.923879532511285));
#13723=DIRECTION('',(-0.336556770590782,-0.475963149477969,0.812519920068743));
#13724=DIRECTION('',(0.,-1.,0.));
#13725=DIRECTION('',(0.336556770590782,-0.475963149477969,-0.812519920068743));
#13726=DIRECTION('',(0.357406744336597,0.357406744336597,-0.862856209461013));
#13727=DIRECTION('center_axis',(0.707106781186548,-0.707106781186548,0.));
#13728=DIRECTION('ref_axis',(0.,0.,-1.));
#13729=DIRECTION('',(-0.707106781186548,-0.707106781186548,-1.57009245868377E-14));
#13730=DIRECTION('',(0.,0.,1.));
#13731=DIRECTION('center_axis',(0.577350269189617,-0.57735026918963,0.57735026918963));
#13732=DIRECTION('ref_axis',(0.707106781186555,0.,-0.70710678118654));
#13733=DIRECTION('',(0.707106781186555,0.,-0.70710678118654));
#13734=DIRECTION('',(0.812519920068752,0.475963149477957,-0.336556770590777));
#13735=DIRECTION('',(0.,0.707106781186548,0.707106781186548));
#13736=DIRECTION('',(-0.475963149477975,0.336556770590777,0.812519920068742));
#13737=DIRECTION('',(-0.812519920068753,-0.336556770590785,0.47596314947795));
#13738=DIRECTION('center_axis',(0.70710678118654,0.,0.707106781186555));
#13739=DIRECTION('ref_axis',(0.707106781186555,0.,-0.70710678118654));
#13740=DIRECTION('',(-0.707106781186555,0.,0.70710678118654));
#13741=DIRECTION('',(0.,1.,0.));
#13742=DIRECTION('center_axis',(0.382683432365087,0.,0.923879532511288));
#13743=DIRECTION('ref_axis',(0.923879532511288,0.,-0.382683432365087));
#13744=DIRECTION('',(-0.812519920068752,0.475963149477957,0.336556770590777));
#13745=DIRECTION('',(-0.862856209461019,-0.357406744336591,0.357406744336591));
#13746=DIRECTION('',(0.,-1.,0.));
#13747=DIRECTION('',(0.862856209461019,-0.357406744336591,-0.357406744336591));
#13748=DIRECTION('center_axis',(0.,-0.707106781186548,0.707106781186548));
#13749=DIRECTION('ref_axis',(1.,0.,0.));
#13750=DIRECTION('',(-1.,0.,0.));
#13751=DIRECTION('',(0.862856209461006,0.357406744336607,0.357406744336607));
#13752=DIRECTION('',(0.,-0.707106781186548,-0.707106781186548));
#13753=DIRECTION('',(-1.,0.,0.));
#13754=DIRECTION('center_axis',(-0.923879532511288,0.,0.382683432365087));
#13755=DIRECTION('ref_axis',(0.382683432365087,0.,0.923879532511288));
#13756=DIRECTION('',(0.336556770590774,0.475963149477971,0.812519920068745));
#13757=DIRECTION('',(0.,1.,0.));
#13758=DIRECTION('',(-0.336556770590774,0.475963149477971,-0.812519920068745));
#13759=DIRECTION('',(-0.357406744336591,-0.357406744336591,-0.862856209461019));
#13760=DIRECTION('',(0.,-1.,0.));
#13761=DIRECTION('',(0.357406744336591,-0.357406744336591,0.862856209461019));
#13762=DIRECTION('center_axis',(-0.577350269189626,-0.577350269189626,0.577350269189626));
#13763=DIRECTION('ref_axis',(0.707106781186548,0.,0.707106781186548));
#13764=DIRECTION('',(-0.707106781186548,0.707106781186548,0.));
#13765=DIRECTION('',(-0.812519920068746,0.336556770590782,-0.475963149477964));
#13766=DIRECTION('',(-0.475963149477967,-0.336556770590779,-0.812519920068746));
#13767=DIRECTION('',(0.812519920068747,-0.475963149477952,0.336556770590795));
#13768=DIRECTION('',(0.707106781186548,0.,0.707106781186548));
#13769=DIRECTION('center_axis',(-0.707106781186548,-0.707106781186548,0.));
#13770=DIRECTION('ref_axis',(0.,0.,1.));
#13771=DIRECTION('',(0.,0.,-1.));
#13772=DIRECTION('',(-0.357406744336594,0.357406744336594,0.862856209461016));
#13773=DIRECTION('',(0.707106781186548,-0.707106781186548,0.));
#13774=DIRECTION('',(0.,0.,-1.));
#13775=DIRECTION('center_axis',(-1.,0.,0.));
#13776=DIRECTION('ref_axis',(0.,0.,1.));
#13777=DIRECTION('',(0.,0.,1.));
#13778=DIRECTION('',(0.,1.,0.));
#13779=DIRECTION('center_axis',(1.,0.,0.));
#13780=DIRECTION('ref_axis',(0.,0.,1.));
#13781=DIRECTION('center_axis',(-0.382683432365106,0.,0.92387953251128));
#13782=DIRECTION('ref_axis',(0.92387953251128,0.,0.382683432365106));
#13783=DIRECTION('',(-0.812519920068747,-0.475963149477952,-0.336556770590795));
#13784=DIRECTION('',(0.,-1.,0.));
#13785=DIRECTION('',(0.,1.,0.));
#13786=DIRECTION('',(-0.862856209461006,0.357406744336607,-0.357406744336607));
#13787=DIRECTION('center_axis',(-0.707106781186548,0.,0.707106781186548));
#13788=DIRECTION('ref_axis',(0.707106781186548,0.,0.707106781186548));
#13789=DIRECTION('',(-0.707106781186548,0.,-0.707106781186548));
#13790=DIRECTION('center_axis',(-0.577350269189626,0.577350269189626,0.577350269189626));
#13791=DIRECTION('ref_axis',(0.707106781186548,0.,0.707106781186548));
#13792=DIRECTION('',(0.,-0.707106781186548,0.707106781186548));
#13793=DIRECTION('',(0.475963149477967,-0.336556770590779,0.812519920068746));
#13794=DIRECTION('',(0.812519920068746,0.336556770590782,0.475963149477964));
#13795=DIRECTION('',(0.707106781186548,0.707106781186548,0.));
#13796=DIRECTION('center_axis',(0.,0.707106781186548,0.707106781186548));
#13797=DIRECTION('ref_axis',(1.,0.,0.));
#13798=DIRECTION('',(0.,0.707106781186548,-0.707106781186548));
#13799=DIRECTION('',(1.,0.,0.));
#13800=DIRECTION('',(1.,0.,0.));
#13801=DIRECTION('center_axis',(-0.923879532511286,0.,-0.382683432365091));
#13802=DIRECTION('ref_axis',(-0.382683432365091,0.,0.923879532511286));
#13803=DIRECTION('',(0.336556770590779,-0.475963149477967,-0.812519920068745));
#13804=DIRECTION('',(0.,-1.,0.));
#13805=DIRECTION('',(-0.336556770590779,-0.475963149477967,0.812519920068745));
#13806=DIRECTION('',(0.357406744336594,0.357406744336594,-0.862856209461016));
#13807=DIRECTION('center_axis',(-0.577350269189626,-0.577350269189626,-0.577350269189626));
#13808=DIRECTION('ref_axis',(-0.707106781186548,0.,0.707106781186547));
#13809=DIRECTION('',(-0.707106781186548,0.,0.707106781186547));
#13810=DIRECTION('',(-0.812519920068746,0.475963149477963,0.336556770590782));
#13811=DIRECTION('',(0.,0.707106781186548,-0.707106781186548));
#13812=DIRECTION('',(0.475963149477967,0.336556770590778,-0.812519920068745));
#13813=DIRECTION('',(0.812519920068746,-0.336556770590782,-0.475963149477963));
#13814=DIRECTION('center_axis',(-0.382683432365094,0.,-0.923879532511285));
#13815=DIRECTION('ref_axis',(-0.923879532511285,0.,0.382683432365094));
#13816=DIRECTION('',(0.,1.,0.));
#13817=DIRECTION('',(0.812519920068746,0.475963149477963,-0.336556770590782));
#13818=DIRECTION('',(0.862856209461014,-0.357406744336597,-0.357406744336597));
#13819=DIRECTION('',(0.,-1.,0.));
#13820=DIRECTION('',(-0.862856209461014,-0.357406744336597,0.357406744336597));
#13821=DIRECTION('center_axis',(0.,0.,-1.));
#13822=DIRECTION('ref_axis',(-1.,0.,0.));
#13823=DIRECTION('',(-1.,0.,0.));
#13824=DIRECTION('',(0.,1.,0.));
#13825=DIRECTION('',(1.,0.,0.));
#13826=DIRECTION('center_axis',(0.,0.707106781186548,-0.707106781186548));
#13827=DIRECTION('ref_axis',(-1.,0.,0.));
#13828=DIRECTION('',(0.,0.707106781186548,0.707106781186548));
#13829=DIRECTION('',(-1.,0.,0.));
#13830=DIRECTION('',(0.,-0.707106781186548,-0.707106781186548));
#13831=DIRECTION('',(0.862856209461015,0.357406744336595,0.357406744336595));
#13832=DIRECTION('center_axis',(-0.577350269189626,0.577350269189626,-0.577350269189626));
#13833=DIRECTION('ref_axis',(-0.707106781186548,0.,0.707106781186547));
#13834=DIRECTION('',(-0.707106781186548,-0.707106781186548,0.));
#13835=DIRECTION('',(-0.812519920068746,-0.336556770590782,0.475963149477963));
#13836=DIRECTION('',(-0.475963149477968,0.336556770590778,0.812519920068745));
#13837=DIRECTION('',(0.707106781186548,0.,-0.707106781186547));
#13838=DIRECTION('center_axis',(0.382683432365092,0.,-0.923879532511286));
#13839=DIRECTION('ref_axis',(-0.923879532511286,0.,-0.382683432365092));
#13840=DIRECTION('',(0.812519920068746,-0.475963149477966,0.33655677059078));
#13841=DIRECTION('',(0.,-1.,0.));
#13842=DIRECTION('',(-0.812519920068746,-0.475963149477966,-0.33655677059078));
#13843=DIRECTION('',(-0.862856209461015,0.357406744336595,-0.357406744336595));
#13844=DIRECTION('center_axis',(0.,-0.707106781186548,-0.707106781186548));
#13845=DIRECTION('ref_axis',(-1.,0.,0.));
#13846=DIRECTION('',(0.,-0.707106781186548,0.707106781186548));
#13847=DIRECTION('',(1.,0.,0.));
#13848=DIRECTION('center_axis',(0.577350269189626,-0.577350269189626,-0.577350269189626));
#13849=DIRECTION('ref_axis',(-0.707106781186548,0.,-0.707106781186548));
#13850=DIRECTION('',(-0.707106781186548,0.,-0.707106781186548));
#13851=DIRECTION('',(-0.336556770590779,0.475963149477967,-0.812519920068746));
#13852=DIRECTION('',(0.707106781186548,0.707106781186548,0.));
#13853=DIRECTION('',(0.812519920068746,0.336556770590778,0.475963149477968));
#13854=DIRECTION('',(0.475963149477967,-0.336556770590778,0.812519920068745));
#13855=DIRECTION('center_axis',(0.923879532511286,0.,-0.382683432365091));
#13856=DIRECTION('ref_axis',(-0.382683432365091,0.,-0.923879532511286));
#13857=DIRECTION('',(0.,1.,0.));
#13858=DIRECTION('',(0.336556770590779,0.475963149477967,0.812519920068746));
#13859=DIRECTION('',(0.357406744336594,-0.357406744336594,0.862856209461016));
#13860=DIRECTION('',(0.,-1.,0.));
#13861=DIRECTION('',(-0.357406744336594,-0.357406744336594,-0.862856209461016));
#13862=DIRECTION('center_axis',(1.,0.,0.));
#13863=DIRECTION('ref_axis',(0.,0.,-1.));
#13864=DIRECTION('',(0.,0.,-1.));
#13865=DIRECTION('center_axis',(1.,0.,0.));
#13866=DIRECTION('ref_axis',(0.,0.707106781186547,-0.707106781186548));
#13867=DIRECTION('',(0.,1.,0.));
#13868=DIRECTION('center_axis',(1.,0.,0.));
#13869=DIRECTION('ref_axis',(0.,-0.707106781186547,-0.707106781186548));
#13870=DIRECTION('',(0.,0.,1.));
#13871=DIRECTION('center_axis',(-1.,0.,0.));
#13872=DIRECTION('ref_axis',(0.,0.,1.));
#13873=DIRECTION('center_axis',(0.707106781186548,0.707106781186548,0.));
#13874=DIRECTION('ref_axis',(0.,0.,-1.));
#13875=DIRECTION('',(-0.707106781186548,0.707106781186548,0.));
#13876=DIRECTION('',(0.,0.,-1.));
#13877=DIRECTION('',(0.707106781186548,-0.707106781186548,0.));
#13878=DIRECTION('center_axis',(0.577350269189626,0.577350269189626,-0.577350269189626));
#13879=DIRECTION('ref_axis',(-0.707106781186548,0.,-0.707106781186548));
#13880=DIRECTION('',(-0.475963149477967,-0.336556770590778,-0.812519920068745));
#13881=DIRECTION('',(-0.812519920068746,0.336556770590778,-0.475963149477968));
#13882=DIRECTION('',(0.707106781186548,0.,0.707106781186548));
#13883=DIRECTION('center_axis',(0.,-0.923879532511287,-0.382683432365091));
#13884=DIRECTION('ref_axis',(0.,0.382683432365091,-0.923879532511287));
#13885=DIRECTION('',(-0.678598344545847,-0.281084637714821,0.678598344545847));
#13886=DIRECTION('',(-1.,0.,0.));
#13887=DIRECTION('',(-0.678598344545843,0.281084637714822,-0.67859834454585));
#13888=DIRECTION('center_axis',(0.38268343236509,-0.923879532511287,0.));
#13889=DIRECTION('ref_axis',(0.,0.,-1.));
#13890=DIRECTION('',(0.,0.,1.));
#13891=DIRECTION('',(0.923879532511287,0.38268343236509,0.));
#13892=DIRECTION('',(0.,0.,-1.));
#13893=DIRECTION('center_axis',(0.,-1.,0.));
#13894=DIRECTION('ref_axis',(0.,0.,-1.));
#13895=DIRECTION('',(-1.,0.,0.));
#13896=DIRECTION('',(0.,0.,1.));
#13897=DIRECTION('',(-1.,0.,0.));
#13898=DIRECTION('',(0.,0.,-1.));
#13899=DIRECTION('',(1.,0.,0.));
#13900=DIRECTION('',(0.,0.,1.));
#13901=DIRECTION('center_axis',(0.,-1.,0.));
#13902=DIRECTION('ref_axis',(1.,0.,0.));
#13903=DIRECTION('center_axis',(0.,-1.,0.));
#13904=DIRECTION('ref_axis',(1.,0.,0.));
#13905=DIRECTION('center_axis',(0.,-1.,0.));
#13906=DIRECTION('ref_axis',(1.,0.,0.));
#13907=DIRECTION('center_axis',(0.,-1.,0.));
#13908=DIRECTION('ref_axis',(1.,0.,0.));
#13909=DIRECTION('',(-0.707106781186548,-0.707106781186548,0.));
#13910=DIRECTION('',(0.71458114110686,0.699552566126676,7.76834820259501E-15));
#13911=DIRECTION('center_axis',(0.,-0.923879532511286,0.382683432365091));
#13912=DIRECTION('ref_axis',(0.,-0.382683432365091,-0.923879532511286));
#13913=DIRECTION('',(0.678598344545843,-0.281084637714822,-0.67859834454585));
#13914=DIRECTION('',(0.678598344545843,0.281084637714822,0.67859834454585));
#13915=DIRECTION('center_axis',(-0.382683432365094,-0.923879532511285,0.));
#13916=DIRECTION('ref_axis',(0.,0.,-1.));
#13917=DIRECTION('center_axis',(0.,-0.923879532511287,-0.382683432365091));
#13918=DIRECTION('ref_axis',(0.,0.382683432365091,-0.923879532511287));
#13919=DIRECTION('',(-0.678598344545843,-0.281084637714822,0.67859834454585));
#13920=DIRECTION('',(-0.678598344545847,0.281084637714821,-0.678598344545847));
#13921=DIRECTION('center_axis',(0.382683432365094,-0.923879532511285,0.));
#13922=DIRECTION('ref_axis',(0.,0.,-1.));
#13923=DIRECTION('center_axis',(-0.38268343236509,-0.923879532511287,0.));
#13924=DIRECTION('ref_axis',(0.,0.,-1.));
#13925=DIRECTION('',(-0.923879532511287,0.38268343236509,0.));
#13926=DIRECTION('center_axis',(0.,0.923879532511287,-0.382683432365091));
#13927=DIRECTION('ref_axis',(0.,0.382683432365091,0.923879532511287));
#13928=DIRECTION('',(0.678598344545847,0.281084637714821,0.678598344545847));
#13929=DIRECTION('',(1.,0.,0.));
#13930=DIRECTION('',(0.678598344545843,-0.281084637714822,-0.67859834454585));
#13931=DIRECTION('center_axis',(-0.38268343236509,0.923879532511287,0.));
#13932=DIRECTION('ref_axis',(0.,0.,1.));
#13933=DIRECTION('',(0.,0.,1.));
#13934=DIRECTION('',(-0.923879532511287,-0.38268343236509,0.));
#13935=DIRECTION('',(0.,0.,-1.));
#13936=DIRECTION('center_axis',(0.,1.,0.));
#13937=DIRECTION('ref_axis',(0.,0.,1.));
#13938=DIRECTION('',(1.,0.,0.));
#13939=DIRECTION('',(0.,0.,1.));
#13940=DIRECTION('',(1.,0.,0.));
#13941=DIRECTION('',(0.,0.,-1.));
#13942=DIRECTION('',(-1.,0.,0.));
#13943=DIRECTION('',(0.,0.,1.));
#13944=DIRECTION('center_axis',(0.,1.,0.));
#13945=DIRECTION('ref_axis',(1.,0.,0.));
#13946=DIRECTION('center_axis',(0.,1.,0.));
#13947=DIRECTION('ref_axis',(1.,0.,0.));
#13948=DIRECTION('center_axis',(0.,1.,0.));
#13949=DIRECTION('ref_axis',(1.,0.,0.));
#13950=DIRECTION('center_axis',(0.,1.,0.));
#13951=DIRECTION('ref_axis',(1.,0.,0.));
#13952=DIRECTION('',(0.707106781186548,0.707106781186548,0.));
#13953=DIRECTION('',(-0.71458114110686,-0.699552566126676,0.));
#13954=DIRECTION('center_axis',(0.,0.923879532511286,0.382683432365091));
#13955=DIRECTION('ref_axis',(0.,-0.382683432365091,0.923879532511286));
#13956=DIRECTION('',(0.475963149477975,0.336556770590777,-0.812519920068742));
#13957=DIRECTION('',(-0.678598344545843,0.281084637714822,-0.67859834454585));
#13958=DIRECTION('',(-0.678598344545843,-0.281084637714822,0.67859834454585));
#13959=DIRECTION('center_axis',(0.382683432365094,0.923879532511285,0.));
#13960=DIRECTION('ref_axis',(0.,0.,1.));
#13961=DIRECTION('',(0.812519920068753,-0.336556770590785,-0.47596314947795));
#13962=DIRECTION('center_axis',(0.577350269189617,0.57735026918963,0.57735026918963));
#13963=DIRECTION('ref_axis',(0.707106781186555,0.,-0.70710678118654));
#13964=DIRECTION('center_axis',(0.,0.923879532511287,-0.382683432365091));
#13965=DIRECTION('ref_axis',(0.,0.382683432365091,0.923879532511287));
#13966=DIRECTION('',(0.678598344545843,0.281084637714822,0.67859834454585));
#13967=DIRECTION('',(0.678598344545847,-0.281084637714821,-0.678598344545847));
#13968=DIRECTION('center_axis',(-0.382683432365094,0.923879532511285,0.));
#13969=DIRECTION('ref_axis',(0.,0.,1.));
#13970=DIRECTION('',(0.,0.,1.));
#13971=DIRECTION('center_axis',(0.38268343236509,0.923879532511287,0.));
#13972=DIRECTION('ref_axis',(0.,0.,1.));
#13973=DIRECTION('',(0.923879532511287,-0.38268343236509,0.));
#13974=DIRECTION('center_axis',(0.,1.,0.));
#13975=DIRECTION('ref_axis',(1.,0.,0.));
#13976=DIRECTION('',(0.707106781186545,-0.70710678118655,-8.6595605623549E-17));
#13977=DIRECTION('center_axis',(0.,-1.,0.));
#13978=DIRECTION('ref_axis',(1.,0.,0.));
#13979=DIRECTION('center_axis',(0.,1.,0.));
#13980=DIRECTION('ref_axis',(1.,0.,0.));
#13981=DIRECTION('center_axis',(0.,1.,0.));
#13982=DIRECTION('ref_axis',(1.,0.,0.));
#13983=DIRECTION('',(0.,1.,0.));
#13984=DIRECTION('center_axis',(0.,-1.,0.));
#13985=DIRECTION('ref_axis',(1.,0.,0.));
#13986=DIRECTION('',(0.707106781186545,0.70710678118655,8.6595605623549E-17));
#13987=DIRECTION('center_axis',(0.,1.,0.));
#13988=DIRECTION('ref_axis',(1.,0.,0.));
#13989=DIRECTION('',(0.707106781186545,-0.70710678118655,-8.6595605623549E-17));
#13990=DIRECTION('center_axis',(0.,-1.,0.));
#13991=DIRECTION('ref_axis',(1.,0.,0.));
#13992=DIRECTION('center_axis',(0.,1.,0.));
#13993=DIRECTION('ref_axis',(1.,0.,0.));
#13994=DIRECTION('center_axis',(0.,1.,0.));
#13995=DIRECTION('ref_axis',(1.,0.,0.));
#13996=DIRECTION('',(0.,1.,0.));
#13997=DIRECTION('center_axis',(0.,-1.,0.));
#13998=DIRECTION('ref_axis',(1.,0.,0.));
#13999=DIRECTION('',(0.707106781186545,0.70710678118655,8.6595605623549E-17));
#14000=DIRECTION('center_axis',(0.,1.,0.));
#14001=DIRECTION('ref_axis',(1.,0.,0.));
#14002=DIRECTION('',(0.707106781186545,-0.70710678118655,-8.6595605623549E-17));
#14003=DIRECTION('center_axis',(0.,-1.,0.));
#14004=DIRECTION('ref_axis',(1.,0.,0.));
#14005=DIRECTION('center_axis',(0.,1.,0.));
#14006=DIRECTION('ref_axis',(1.,0.,0.));
#14007=DIRECTION('center_axis',(0.,1.,0.));
#14008=DIRECTION('ref_axis',(1.,0.,0.));
#14009=DIRECTION('',(0.,1.,0.));
#14010=DIRECTION('center_axis',(0.,-1.,0.));
#14011=DIRECTION('ref_axis',(1.,0.,0.));
#14012=DIRECTION('',(0.707106781186545,0.70710678118655,8.6595605623549E-17));
#14013=DIRECTION('center_axis',(0.,1.,0.));
#14014=DIRECTION('ref_axis',(1.,0.,0.));
#14015=DIRECTION('',(0.707106781186545,-0.70710678118655,-8.6595605623549E-17));
#14016=DIRECTION('center_axis',(0.,-1.,0.));
#14017=DIRECTION('ref_axis',(1.,0.,0.));
#14018=DIRECTION('center_axis',(0.,1.,0.));
#14019=DIRECTION('ref_axis',(1.,0.,0.));
#14020=DIRECTION('center_axis',(0.,1.,0.));
#14021=DIRECTION('ref_axis',(1.,0.,0.));
#14022=DIRECTION('',(0.,1.,0.));
#14023=DIRECTION('center_axis',(0.,-1.,0.));
#14024=DIRECTION('ref_axis',(1.,0.,0.));
#14025=DIRECTION('',(0.707106781186545,0.70710678118655,8.6595605623549E-17));
#14026=DIRECTION('center_axis',(0.,0.,-1.));
#14027=DIRECTION('ref_axis',(1.,0.,0.));
#14028=DIRECTION('center_axis',(0.,0.,1.));
#14029=DIRECTION('ref_axis',(1.,0.,0.));
#14030=DIRECTION('',(0.707106781186548,8.65956056235494E-17,0.707106781186547));
#14031=DIRECTION('center_axis',(0.,0.,1.));
#14032=DIRECTION('ref_axis',(1.,0.,0.));
#14033=DIRECTION('center_axis',(0.,0.,1.));
#14034=DIRECTION('ref_axis',(1.,0.,0.));
#14035=DIRECTION('',(0.,0.,1.));
#14036=DIRECTION('center_axis',(0.,0.,1.));
#14037=DIRECTION('ref_axis',(1.,0.,0.));
#14038=DIRECTION('center_axis',(0.,0.,1.));
#14039=DIRECTION('ref_axis',(1.,0.,0.));
#14040=DIRECTION('center_axis',(0.,0.,1.));
#14041=DIRECTION('ref_axis',(1.,0.,0.));
#14042=DIRECTION('center_axis',(0.,0.,1.));
#14043=DIRECTION('ref_axis',(1.,0.,0.));
#14044=DIRECTION('',(0.,0.,1.));
#14045=DIRECTION('center_axis',(0.,0.,1.));
#14046=DIRECTION('ref_axis',(1.,0.,0.));
#14047=DIRECTION('center_axis',(0.,0.,-1.));
#14048=DIRECTION('ref_axis',(-1.,0.,0.));
#14049=DIRECTION('center_axis',(0.,0.,1.));
#14050=DIRECTION('ref_axis',(1.,0.,0.));
#14051=DIRECTION('center_axis',(0.,0.,1.));
#14052=DIRECTION('ref_axis',(1.,0.,0.));
#14053=DIRECTION('',(0.,0.,1.));
#14054=DIRECTION('center_axis',(0.,0.,1.));
#14055=DIRECTION('ref_axis',(1.,0.,0.));
#14056=DIRECTION('center_axis',(0.,0.,1.));
#14057=DIRECTION('ref_axis',(1.,0.,0.));
#14058=DIRECTION('',(-0.707106781186542,-8.65956056235487E-17,0.707106781186553));
#14059=DIRECTION('center_axis',(0.,0.,-1.));
#14060=DIRECTION('ref_axis',(1.,0.,0.));
#14061=DIRECTION('center_axis',(1.,0.,0.));
#14062=DIRECTION('ref_axis',(0.,0.,1.));
#14063=DIRECTION('',(-0.707106781186546,8.65956056235495E-17,0.707106781186549));
#14064=DIRECTION('center_axis',(-1.,0.,0.));
#14065=DIRECTION('ref_axis',(0.,0.,1.));
#14066=DIRECTION('center_axis',(-1.,0.,0.));
#14067=DIRECTION('ref_axis',(0.,0.,1.));
#14068=DIRECTION('',(-1.,0.,0.));
#14069=DIRECTION('center_axis',(-1.,0.,0.));
#14070=DIRECTION('ref_axis',(0.,0.,1.));
#14071=DIRECTION('center_axis',(-1.,0.,0.));
#14072=DIRECTION('ref_axis',(0.,0.,1.));
#14073=DIRECTION('center_axis',(-1.,0.,0.));
#14074=DIRECTION('ref_axis',(0.,0.,1.));
#14075=DIRECTION('center_axis',(-1.,0.,0.));
#14076=DIRECTION('ref_axis',(0.,0.,1.));
#14077=DIRECTION('',(-1.,0.,0.));
#14078=DIRECTION('center_axis',(-1.,0.,0.));
#14079=DIRECTION('ref_axis',(0.,0.,1.));
#14080=DIRECTION('center_axis',(1.,0.,0.));
#14081=DIRECTION('ref_axis',(0.,0.,-1.));
#14082=DIRECTION('center_axis',(-1.,0.,0.));
#14083=DIRECTION('ref_axis',(0.,0.,1.));
#14084=DIRECTION('center_axis',(-1.,0.,0.));
#14085=DIRECTION('ref_axis',(0.,0.,1.));
#14086=DIRECTION('',(-1.,0.,0.));
#14087=DIRECTION('center_axis',(-1.,0.,0.));
#14088=DIRECTION('ref_axis',(0.,0.,1.));
#14089=DIRECTION('center_axis',(-1.,0.,0.));
#14090=DIRECTION('ref_axis',(0.,0.,1.));
#14091=DIRECTION('',(-0.707106781186544,-8.65956056235497E-17,-0.707106781186551));
#14092=DIRECTION('center_axis',(1.,0.,0.));
#14093=DIRECTION('ref_axis',(0.,0.,1.));
#14094=DIRECTION('',(-0.707106781186544,8.65956056235497E-17,0.707106781186551));
#14095=DIRECTION('center_axis',(-1.,0.,0.));
#14096=DIRECTION('ref_axis',(0.,0.,1.));
#14097=DIRECTION('center_axis',(-1.,0.,0.));
#14098=DIRECTION('ref_axis',(0.,0.,1.));
#14099=DIRECTION('',(-1.,0.,0.));
#14100=DIRECTION('center_axis',(-1.,0.,0.));
#14101=DIRECTION('ref_axis',(0.,0.,1.));
#14102=DIRECTION('center_axis',(-1.,0.,0.));
#14103=DIRECTION('ref_axis',(0.,0.,1.));
#14104=DIRECTION('center_axis',(-1.,0.,0.));
#14105=DIRECTION('ref_axis',(0.,0.,1.));
#14106=DIRECTION('center_axis',(-1.,0.,0.));
#14107=DIRECTION('ref_axis',(0.,0.,1.));
#14108=DIRECTION('',(-1.,0.,0.));
#14109=DIRECTION('center_axis',(-1.,0.,0.));
#14110=DIRECTION('ref_axis',(0.,0.,1.));
#14111=DIRECTION('center_axis',(1.,0.,0.));
#14112=DIRECTION('ref_axis',(0.,0.,-1.));
#14113=DIRECTION('center_axis',(-1.,0.,0.));
#14114=DIRECTION('ref_axis',(0.,0.,1.));
#14115=DIRECTION('center_axis',(-1.,0.,0.));
#14116=DIRECTION('ref_axis',(0.,0.,1.));
#14117=DIRECTION('',(-1.,0.,0.));
#14118=DIRECTION('center_axis',(-1.,0.,0.));
#14119=DIRECTION('ref_axis',(0.,0.,1.));
#14120=DIRECTION('center_axis',(-1.,0.,0.));
#14121=DIRECTION('ref_axis',(0.,0.,1.));
#14122=DIRECTION('',(-0.707106781186546,-8.65956056235495E-17,-0.707106781186549));
#14123=DIRECTION('center_axis',(0.707106781186548,0.,-0.707106781186548));
#14124=DIRECTION('ref_axis',(-0.707106781186548,0.,-0.707106781186548));
#14125=DIRECTION('center_axis',(-0.707106781186547,0.,-0.707106781186548));
#14126=DIRECTION('ref_axis',(-0.707106781186548,0.,0.707106781186547));
#14127=DIRECTION('center_axis',(0.707106781186548,0.,-0.707106781186548));
#14128=DIRECTION('ref_axis',(-0.707106781186548,0.,-0.707106781186548));
#14129=DIRECTION('center_axis',(-0.707106781186547,0.,-0.707106781186548));
#14130=DIRECTION('ref_axis',(-0.707106781186548,0.,0.707106781186547));
#14131=DIRECTION('center_axis',(-0.707106781186548,0.707106781186548,0.));
#14132=DIRECTION('ref_axis',(0.,0.,1.));
#14133=DIRECTION('center_axis',(-0.707106781186548,0.707106781186548,0.));
#14134=DIRECTION('ref_axis',(0.,0.,1.));
#14135=DIRECTION('center_axis',(0.707106781186548,-0.707106781186548,0.));
#14136=DIRECTION('ref_axis',(0.,0.,-1.));
#14137=DIRECTION('',(0.714581141106858,-0.699552566126678,0.));
#14138=DIRECTION('',(-0.714581141106858,0.699552566126678,0.));
#14139=DIRECTION('center_axis',(1.,0.,0.));
#14140=DIRECTION('ref_axis',(0.,0.,-1.));
#14141=DIRECTION('center_axis',(0.,1.,0.));
#14142=DIRECTION('ref_axis',(-1.,0.,0.));
#14143=DIRECTION('center_axis',(-1.,0.,0.));
#14144=DIRECTION('ref_axis',(0.,-0.707106781186547,-0.707106781186548));
#14145=DIRECTION('center_axis',(1.,0.,0.));
#14146=DIRECTION('ref_axis',(0.,0.,-1.));
#14147=DIRECTION('center_axis',(-1.,0.,0.));
#14148=DIRECTION('ref_axis',(0.,0.707106781186547,-0.707106781186548));
#14149=DIRECTION('center_axis',(0.,1.,0.));
#14150=DIRECTION('ref_axis',(-1.,0.,0.));
#14151=DIRECTION('center_axis',(0.,0.,1.));
#14152=DIRECTION('ref_axis',(1.,0.,0.));
#14153=DIRECTION('center_axis',(-1.,0.,0.));
#14154=DIRECTION('ref_axis',(0.,0.,1.));
#14155=DIRECTION('center_axis',(0.,-1.,0.));
#14156=DIRECTION('ref_axis',(1.,0.,0.));
#14157=DIRECTION('center_axis',(1.,0.,0.));
#14158=DIRECTION('ref_axis',(0.,0.707106781186547,-0.707106781186548));
#14159=DIRECTION('center_axis',(0.,1.,0.));
#14160=DIRECTION('ref_axis',(0.707106781186547,0.,0.707106781186547));
#14161=DIRECTION('center_axis',(0.,-1.,0.));
#14162=DIRECTION('ref_axis',(1.,0.,0.));
#14163=DIRECTION('',(0.,1.,0.));
#14164=DIRECTION('center_axis',(-1.,0.,0.));
#14165=DIRECTION('ref_axis',(0.,0.,1.));
#14166=DIRECTION('center_axis',(1.,0.,0.));
#14167=DIRECTION('ref_axis',(0.,-0.707106781186547,-0.707106781186548));
#14168=DIRECTION('center_axis',(0.,1.,0.));
#14169=DIRECTION('ref_axis',(-0.707106781186547,0.,0.707106781186547));
#14170=DIRECTION('',(0.,-1.,0.));
#14171=DIRECTION('center_axis',(-1.,0.,0.));
#14172=DIRECTION('ref_axis',(0.,0.707106781186547,-0.707106781186547));
#14173=DIRECTION('',(-1.,0.,0.));
#14174=DIRECTION('center_axis',(0.,0.,-1.));
#14175=DIRECTION('ref_axis',(-1.,0.,0.));
#14176=DIRECTION('',(1.,0.,0.));
#14177=DIRECTION('center_axis',(1.,0.,0.));
#14178=DIRECTION('ref_axis',(0.,-0.707106781186547,-0.707106781186547));
#16340=CARTESIAN_POINT('',(0.,0.,0.));
#16341=CARTESIAN_POINT('Origin',(2.71767766952966,0.,0.0873223304703366));
#16342=CARTESIAN_POINT('',(2.72071067811865,2.54071067811865,0.0800000000000001));
#16343=CARTESIAN_POINT('',(2.73535533905933,2.52,0.0446446609406728));
#16344=CARTESIAN_POINT('',(2.92352004688311,2.25389491823563,-0.409625128647481));
#16345=CARTESIAN_POINT('',(2.73535533905933,-2.52,0.0446446609406728));
#16346=CARTESIAN_POINT('',(2.73535533905933,0.,0.0446446609406729));
#16347=CARTESIAN_POINT('',(2.72071067811865,-2.54071067811865,0.0800000000000001));
#16348=CARTESIAN_POINT('',(2.93898922848989,-2.23201819180851,-0.446971036681382));
#16349=CARTESIAN_POINT('',(2.7,-2.52,0.13));
#16350=CARTESIAN_POINT('',(2.23461061779379,-2.05461061779379,1.25354935830668));
#16351=CARTESIAN_POINT('',(2.7,2.52,0.13));
#16352=CARTESIAN_POINT('',(2.7,0.,0.13));
#16353=CARTESIAN_POINT('',(2.23461061779379,2.05461061779379,1.25354935830668));
#16354=CARTESIAN_POINT('Origin',(2.7,0.,0.));
#16355=CARTESIAN_POINT('',(2.7,-2.52,5.36678788880707));
#16356=CARTESIAN_POINT('',(2.7,-2.52,2.1875));
#16357=CARTESIAN_POINT('',(2.7,-2.2,5.3));
#16358=CARTESIAN_POINT('Origin',(2.7,-2.2,6.1));
#16359=CARTESIAN_POINT('',(2.7,2.2,5.3));
#16360=CARTESIAN_POINT('',(2.7,0.,5.3));
#16361=CARTESIAN_POINT('',(2.7,2.52,5.36678788880707));
#16362=CARTESIAN_POINT('Origin',(2.7,2.2,6.1));
#16363=CARTESIAN_POINT('',(2.7,2.52,2.1875));
#16364=CARTESIAN_POINT('',(2.7,1.65327317884893E-16,1.65));
#16365=CARTESIAN_POINT('Origin',(2.7,0.,3.));
#16366=CARTESIAN_POINT('Origin',(2.74,-2.56,2.1875));
#16367=CARTESIAN_POINT('',(2.74464466094067,-2.56464466094067,0.0800000000000001));
#16368=CARTESIAN_POINT('',(2.7,-2.52,0.0800000000000001));
#16369=CARTESIAN_POINT('',(2.74464466094067,-2.56464466094067,5.36678788880707));
#16370=CARTESIAN_POINT('',(2.74464466094067,-2.56464466094067,3.28125));
#16371=CARTESIAN_POINT('',(2.78,-2.6,5.36678788880707));
#16372=CARTESIAN_POINT('Origin',(2.78,-2.52,0.));
#16373=CARTESIAN_POINT('',(2.74464466094067,-2.52,0.0353553390593272));
#16374=CARTESIAN_POINT('',(2.78,-2.52,0.));
#16375=CARTESIAN_POINT('',(2.78,-2.54071067811865,0.0207106781186547));
#16376=CARTESIAN_POINT('',(2.29037487135252,-2.25389491823563,0.223520046883111));
#16377=CARTESIAN_POINT('',(2.78,-2.56464466094067,0.0446446609406727));
#16378=CARTESIAN_POINT('',(2.78,-2.6,0.0800000000000001));
#16379=CARTESIAN_POINT('',(2.76693980625181,-2.57387961250363,0.0669398062518134));
#16380=CARTESIAN_POINT('',(2.63047465709621,-2.67037504486719,0.299900387770978));
#16381=CARTESIAN_POINT('',(2.1631759401255,-2.32379243068329,0.420616490557792));
#16382=CARTESIAN_POINT('Origin',(2.78732233047034,0.,0.0176776695296635));
#16383=CARTESIAN_POINT('',(2.74464466094067,2.52,0.0353553390593272));
#16384=CARTESIAN_POINT('',(2.74464466094067,0.,0.0353553390593271));
#16385=CARTESIAN_POINT('',(2.78,2.54071067811865,0.0207106781186547));
#16386=CARTESIAN_POINT('',(2.25302896331862,2.23201819180851,0.238989228489892));
#16387=CARTESIAN_POINT('',(2.83,2.52,0.));
#16388=CARTESIAN_POINT('',(3.20437526486246,2.36492868787695,-0.155071312123047));
#16389=CARTESIAN_POINT('',(2.83,-2.52,0.));
#16390=CARTESIAN_POINT('',(2.83,0.,0.));
#16391=CARTESIAN_POINT('',(3.20437526486246,-2.36492868787695,-0.155071312123047));
#16392=CARTESIAN_POINT('Origin',(5.75,0.,0.));
#16393=CARTESIAN_POINT('',(5.62,2.52,0.));
#16394=CARTESIAN_POINT('',(2.875,2.52,0.));
#16395=CARTESIAN_POINT('',(5.62,-2.52,0.));
#16396=CARTESIAN_POINT('',(5.62,0.,0.));
#16397=CARTESIAN_POINT('',(2.875,-2.52,0.));
#16398=CARTESIAN_POINT('Origin',(2.875,2.56,0.04));
#16399=CARTESIAN_POINT('',(2.78,2.56464466094067,0.0446446609406727));
#16400=CARTESIAN_POINT('',(2.78,2.52,0.));
#16401=CARTESIAN_POINT('',(5.67,2.56464466094067,0.0446446609406727));
#16402=CARTESIAN_POINT('',(1.4375,2.56464466094067,0.0446446609406726));
#16403=CARTESIAN_POINT('',(5.67,2.54071067811865,0.0207106781186545));
#16404=CARTESIAN_POINT('',(5.67,2.6,0.0800000000000001));
#16405=CARTESIAN_POINT('',(4.24052160356021,1.94860133919395,-0.571398660806053));
#16406=CARTESIAN_POINT('Origin',(2.7,2.52,0.08));
#16407=CARTESIAN_POINT('',(2.74464466094067,2.56464466094067,0.0800000000000001));
#16408=CARTESIAN_POINT('',(2.78,2.6,0.0800000000000001));
#16409=CARTESIAN_POINT('',(2.76693980625181,2.57387961250363,0.0669398062518132));
#16410=CARTESIAN_POINT('',(2.12129921369838,2.30644652264939,0.445147308951012));
#16411=CARTESIAN_POINT('',(2.60594383870299,2.68772095290109,0.3417771141981));
#16412=CARTESIAN_POINT('',(2.7,2.52,0.08));
#16413=CARTESIAN_POINT('Origin',(5.66267766952966,0.,0.0176776695296637));
#16414=CARTESIAN_POINT('',(5.70535533905933,2.52,0.0353553390593273));
#16415=CARTESIAN_POINT('',(6.15962512864748,2.25389491823563,0.223520046883112));
#16416=CARTESIAN_POINT('',(5.70535533905933,-2.52,0.0353553390593273));
#16417=CARTESIAN_POINT('',(5.70535533905933,0.,0.0353553390593273));
#16418=CARTESIAN_POINT('',(5.67,-2.54071067811865,0.0207106781186545));
#16419=CARTESIAN_POINT('',(6.19697103668138,-2.23201819180851,0.238989228489893));
#16420=CARTESIAN_POINT('',(4.24052160356021,-1.94860133919395,-0.571398660806053));
#16421=CARTESIAN_POINT('Origin',(2.875,-2.56,0.04));
#16422=CARTESIAN_POINT('',(5.67,-2.56464466094067,0.0446446609406727));
#16423=CARTESIAN_POINT('',(5.67,-2.52,0.));
#16424=CARTESIAN_POINT('',(1.4375,-2.56464466094067,0.0446446609406726));
#16425=CARTESIAN_POINT('Origin',(5.75,-2.52,0.0800000000000001));
#16426=CARTESIAN_POINT('',(5.71464466094067,-2.52,0.0446446609406718));
#16427=CARTESIAN_POINT('',(5.75,-2.52,0.0800000000000001));
#16428=CARTESIAN_POINT('',(5.72928932188135,-2.54071067811866,0.0800000000000001));
#16429=CARTESIAN_POINT('',(5.52647995311688,-2.25389491823565,-0.409625128647469));
#16430=CARTESIAN_POINT('',(5.70535533905933,-2.56464466094067,0.0800000000000001));
#16431=CARTESIAN_POINT('',(5.67,-2.6,0.0800000000000001));
#16432=CARTESIAN_POINT('',(5.68306019374819,-2.57387961250363,0.0669398062518129));
#16433=CARTESIAN_POINT('',(6.75168622086201,-2.1312402189682,0.692926439830206));
#16434=CARTESIAN_POINT('',(5.21257334774201,-2.24119517323359,-0.736231479024399));
#16435=CARTESIAN_POINT('Origin',(5.73232233047034,0.,0.0873223304703347));
#16436=CARTESIAN_POINT('',(5.71464466094067,2.52,0.0446446609406718));
#16437=CARTESIAN_POINT('',(5.71464466094067,0.,0.0446446609406716));
#16438=CARTESIAN_POINT('',(5.72928932188135,2.54071067811866,0.0800000000000001));
#16439=CARTESIAN_POINT('',(5.5110107715101,2.23201819180853,-0.446971036681371));
#16440=CARTESIAN_POINT('',(5.75,2.52,0.129999999999997));
#16441=CARTESIAN_POINT('',(6.88999388238703,1.38000611761297,2.88218869188102));
#16442=CARTESIAN_POINT('',(5.75,-2.52,0.129999999999997));
#16443=CARTESIAN_POINT('',(5.75,0.,0.129999999999998));
#16444=CARTESIAN_POINT('',(6.88999388238703,-1.38000611761297,2.88218869188102));
#16445=CARTESIAN_POINT('Origin',(5.75,0.,8.75));
#16446=CARTESIAN_POINT('',(5.75,2.52,8.62));
#16447=CARTESIAN_POINT('',(5.75,2.52,6.5625));
#16448=CARTESIAN_POINT('',(5.75,-2.52,8.62));
#16449=CARTESIAN_POINT('',(5.75,0.,8.62));
#16450=CARTESIAN_POINT('',(5.75,-2.52,6.5625));
#16451=CARTESIAN_POINT('',(5.75,-1.65327317884893E-16,1.65));
#16452=CARTESIAN_POINT('Origin',(5.75,0.,3.));
#16453=CARTESIAN_POINT('Origin',(5.71,2.56,6.5625));
#16454=CARTESIAN_POINT('',(5.70535533905933,2.56464466094067,0.0800000000000001));
#16455=CARTESIAN_POINT('',(5.75,2.52,0.0800000000000001));
#16456=CARTESIAN_POINT('',(5.70535533905933,2.56464466094067,8.67));
#16457=CARTESIAN_POINT('',(5.70535533905933,2.56464466094067,5.46875));
#16458=CARTESIAN_POINT('',(5.72928932188134,2.54071067811866,8.67));
#16459=CARTESIAN_POINT('',(5.67,2.6,8.67));
#16460=CARTESIAN_POINT('',(6.21538938220622,2.05461061779378,7.49645064169333));
#16461=CARTESIAN_POINT('Origin',(5.67,2.52,0.));
#16462=CARTESIAN_POINT('',(5.68306019374819,2.57387961250363,0.0669398062518126));
#16463=CARTESIAN_POINT('',(5.18804252934879,2.22384926519969,-0.77810820545152));
#16464=CARTESIAN_POINT('',(6.70980949443489,2.1485861270021,0.668395621436986));
#16465=CARTESIAN_POINT('',(5.67,2.52,0.));
#16466=CARTESIAN_POINT('Origin',(5.73232233047034,0.,8.66267766952966));
#16467=CARTESIAN_POINT('',(5.71464466094067,2.52,8.70535533905933));
#16468=CARTESIAN_POINT('',(5.52647995311688,2.25389491823563,9.15962512864748));
#16469=CARTESIAN_POINT('',(5.71464466094067,-2.52,8.70535533905933));
#16470=CARTESIAN_POINT('',(5.71464466094067,0.,8.70535533905933));
#16471=CARTESIAN_POINT('',(5.72928932188134,-2.54071067811866,8.67));
#16472=CARTESIAN_POINT('',(5.5110107715101,-2.23201819180851,9.19697103668138));
#16473=CARTESIAN_POINT('',(6.21538938220622,-2.05461061779378,7.49645064169333));
#16474=CARTESIAN_POINT('Origin',(5.71,-2.56,6.5625));
#16475=CARTESIAN_POINT('',(5.70535533905933,-2.56464466094067,8.67));
#16476=CARTESIAN_POINT('',(5.75,-2.52,8.67));
#16477=CARTESIAN_POINT('',(5.70535533905933,-2.56464466094067,5.46875));
#16478=CARTESIAN_POINT('Origin',(5.67,-2.52,8.75));
#16479=CARTESIAN_POINT('',(5.70535533905933,-2.52,8.71464466094067));
#16480=CARTESIAN_POINT('',(5.67,-2.52,8.75));
#16481=CARTESIAN_POINT('',(5.67,-2.54071067811866,8.72928932188134));
#16482=CARTESIAN_POINT('',(6.15962512864747,-2.25389491823565,8.52647995311689));
#16483=CARTESIAN_POINT('',(5.67,-2.56464466094067,8.70535533905933));
#16484=CARTESIAN_POINT('',(5.67,-2.6,8.67));
#16485=CARTESIAN_POINT('',(5.68306019374819,-2.57387961250363,8.68306019374819));
#16486=CARTESIAN_POINT('',(4.8623899573361,-1.99357812321868,10.0840319194452));
#16487=CARTESIAN_POINT('',(6.28682405987448,-2.3237924306833,8.32938350944224));
#16488=CARTESIAN_POINT('Origin',(5.71,0.,8.71));
#16489=CARTESIAN_POINT('',(5.70535533905933,2.52,8.71464466094067));
#16490=CARTESIAN_POINT('',(5.75,2.52,8.67));
#16491=CARTESIAN_POINT('',(5.70535533905933,0.,8.71464466094067));
#16492=CARTESIAN_POINT('Origin',(5.66267766952966,0.,8.73232233047034));
#16493=CARTESIAN_POINT('',(5.67,2.54071067811866,8.72928932188134));
#16494=CARTESIAN_POINT('',(6.19697103668137,2.23201819180853,8.51101077151011));
#16495=CARTESIAN_POINT('',(5.62,2.52,8.75));
#16496=CARTESIAN_POINT('',(2.10002419371957,1.06197828181349,10.2080217181865));
#16497=CARTESIAN_POINT('',(5.62,-2.52,8.75));
#16498=CARTESIAN_POINT('',(5.62,0.,8.75));
#16499=CARTESIAN_POINT('',(2.10002419371957,-1.06197828181349,10.2080217181865));
#16500=CARTESIAN_POINT('Origin',(-2.875,-2.56,8.71));
#16501=CARTESIAN_POINT('',(-5.62,-2.52,8.75));
#16502=CARTESIAN_POINT('',(-2.875,-2.52,8.75));
#16503=CARTESIAN_POINT('',(-5.67,-2.54071067811865,8.72928932188134));
#16504=CARTESIAN_POINT('',(-4.24052160356022,-1.94860133919393,9.32139866080608));
#16505=CARTESIAN_POINT('',(-5.67,-2.56464466094067,8.70535533905933));
#16506=CARTESIAN_POINT('',(-5.67,-2.52,8.75));
#16507=CARTESIAN_POINT('',(-1.4375,-2.56464466094067,8.70535533905933));
#16508=CARTESIAN_POINT('Origin',(-5.73232233047034,0.,8.66267766952966));
#16509=CARTESIAN_POINT('',(-5.72928932188135,-2.54071067811865,8.67));
#16510=CARTESIAN_POINT('',(-5.71464466094067,-2.52,8.70535533905933));
#16511=CARTESIAN_POINT('',(-5.52647995311689,-2.25389491823563,9.15962512864748));
#16512=CARTESIAN_POINT('',(-5.71464466094067,2.52,8.70535533905933));
#16513=CARTESIAN_POINT('',(-5.71464466094067,0.,8.70535533905933));
#16514=CARTESIAN_POINT('',(-5.72928932188135,2.54071067811865,8.67));
#16515=CARTESIAN_POINT('',(-5.51101077151011,2.23201819180851,9.19697103668138));
#16516=CARTESIAN_POINT('',(-5.75,2.52,8.62));
#16517=CARTESIAN_POINT('',(-6.889993882387,1.380006117613,5.86781130811893));
#16518=CARTESIAN_POINT('',(-5.75,-2.52,8.62));
#16519=CARTESIAN_POINT('',(-5.75,0.,8.62));
#16520=CARTESIAN_POINT('',(-6.889993882387,-1.380006117613,5.86781130811893));
#16521=CARTESIAN_POINT('Origin',(-5.75,-2.52,8.67));
#16522=CARTESIAN_POINT('',(-5.70535533905933,-2.56464466094067,8.67));
#16523=CARTESIAN_POINT('',(-5.67,-2.6,8.67));
#16524=CARTESIAN_POINT('',(-5.68306019374819,-2.57387961250363,8.68306019374819));
#16525=CARTESIAN_POINT('',(-6.75168622086201,-2.1312402189682,8.05707356016979));
#16526=CARTESIAN_POINT('',(-5.21257334774201,-2.24119517323359,9.4862314790244));
#16527=CARTESIAN_POINT('',(-5.70535533905933,-2.52,8.71464466094067));
#16528=CARTESIAN_POINT('',(-6.19697103668137,-2.23201819180853,8.5110107715101));
#16529=CARTESIAN_POINT('',(-5.75,-2.52,8.67));
#16530=CARTESIAN_POINT('Origin',(-5.71,-2.56,2.1875));
#16531=CARTESIAN_POINT('',(-5.75,-2.52,0.129999999999999));
#16532=CARTESIAN_POINT('',(-5.75,-2.52,2.1875));
#16533=CARTESIAN_POINT('',(-5.72928932188135,-2.54071067811865,0.0800000000000001));
#16534=CARTESIAN_POINT('',(-6.21538938220622,-2.05461061779379,1.25354935830668));
#16535=CARTESIAN_POINT('',(-5.70535533905933,-2.56464466094067,0.0800000000000001));
#16536=CARTESIAN_POINT('',(-5.75,-2.52,0.0800000000000001));
#16537=CARTESIAN_POINT('',(-5.70535533905933,-2.56464466094067,3.28125));
#16538=CARTESIAN_POINT('Origin',(-5.75,0.,0.));
#16539=CARTESIAN_POINT('',(-5.75,2.52,0.129999999999999));
#16540=CARTESIAN_POINT('',(-5.75,2.52,2.1875));
#16541=CARTESIAN_POINT('',(-5.75,0.,0.129999999999999));
#16542=CARTESIAN_POINT('',(-5.75,1.65327317884893E-16,1.65));
#16543=CARTESIAN_POINT('Origin',(-5.75,0.,3.));
#16544=CARTESIAN_POINT('Origin',(-5.66267766952967,0.,8.73232233047034));
#16545=CARTESIAN_POINT('',(-5.67,2.54071067811865,8.72928932188134));
#16546=CARTESIAN_POINT('',(-5.70535533905933,2.52,8.71464466094067));
#16547=CARTESIAN_POINT('',(-6.15962512864747,2.25389491823565,8.52647995311688));
#16548=CARTESIAN_POINT('',(-5.70535533905933,0.,8.71464466094067));
#16549=CARTESIAN_POINT('',(-5.62,2.52,8.75));
#16550=CARTESIAN_POINT('',(-5.62,0.,8.75));
#16551=CARTESIAN_POINT('',(-4.24052160356022,1.94860133919393,9.32139866080608));
#16552=CARTESIAN_POINT('Origin',(-5.71,0.,8.71));
#16553=CARTESIAN_POINT('',(-5.67,2.52,8.75));
#16554=CARTESIAN_POINT('Origin',(-5.67,2.52,8.75));
#16555=CARTESIAN_POINT('',(-5.67,2.56464466094067,8.70535533905933));
#16556=CARTESIAN_POINT('',(-5.67,2.6,8.67));
#16557=CARTESIAN_POINT('',(-5.68306019374819,2.57387961250363,8.68306019374819));
#16558=CARTESIAN_POINT('',(-5.18804252934879,2.22384926519969,9.52810820545152));
#16559=CARTESIAN_POINT('',(-5.70535533905933,2.56464466094067,8.67));
#16560=CARTESIAN_POINT('',(-6.70980949443489,2.1485861270021,8.08160437856301));
#16561=CARTESIAN_POINT('',(-5.75,2.52,8.67));
#16562=CARTESIAN_POINT('Origin',(-2.875,2.56,8.71));
#16563=CARTESIAN_POINT('',(5.67,2.56464466094067,8.70535533905933));
#16564=CARTESIAN_POINT('',(5.67,2.52,8.75));
#16565=CARTESIAN_POINT('',(-1.4375,2.56464466094067,8.70535533905933));
#16566=CARTESIAN_POINT('',(-2.875,2.52,8.75));
#16567=CARTESIAN_POINT('Origin',(-5.73232233047034,0.,0.0873223304703359));
#16568=CARTESIAN_POINT('',(-5.72928932188135,2.54071067811865,0.0800000000000001));
#16569=CARTESIAN_POINT('',(-5.71464466094067,2.52,0.0446446609406726));
#16570=CARTESIAN_POINT('',(-5.52647995311689,2.25389491823563,-0.409625128647479));
#16571=CARTESIAN_POINT('',(-5.71464466094067,-2.52,0.0446446609406726));
#16572=CARTESIAN_POINT('',(-5.71464466094067,0.,0.0446446609406725));
#16573=CARTESIAN_POINT('',(-5.51101077151011,-2.23201819180851,-0.44697103668138));
#16574=CARTESIAN_POINT('',(-6.21538938220622,2.05461061779379,1.25354935830668));
#16575=CARTESIAN_POINT('Origin',(-5.67,-2.52,0.));
#16576=CARTESIAN_POINT('',(-5.70535533905933,-2.52,0.035355339059328));
#16577=CARTESIAN_POINT('',(-5.67,-2.52,0.));
#16578=CARTESIAN_POINT('',(-5.67,-2.54071067811865,0.0207106781186548));
#16579=CARTESIAN_POINT('',(-6.15962512864748,-2.25389491823564,0.223520046883113));
#16580=CARTESIAN_POINT('',(-5.67,-2.56464466094067,0.0446446609406727));
#16581=CARTESIAN_POINT('',(-5.67,-2.6,0.0800000000000001));
#16582=CARTESIAN_POINT('',(-5.68306019374819,-2.57387961250363,0.0669398062518126));
#16583=CARTESIAN_POINT('',(-5.10167380372804,-2.16277735363081,-0.925548842641145));
#16584=CARTESIAN_POINT('',(-6.28682405987449,-2.32379243068329,0.420616490557785));
#16585=CARTESIAN_POINT('Origin',(-5.66267766952966,0.,0.0176776695296639));
#16586=CARTESIAN_POINT('',(-5.70535533905933,2.52,0.035355339059328));
#16587=CARTESIAN_POINT('',(-5.70535533905933,0.,0.0353553390593278));
#16588=CARTESIAN_POINT('',(-5.67,2.54071067811865,0.0207106781186548));
#16589=CARTESIAN_POINT('',(-6.19697103668138,2.23201819180852,0.238989228489894));
#16590=CARTESIAN_POINT('',(-5.62,2.52,0.));
#16591=CARTESIAN_POINT('',(-3.67282446442857,1.71345348484521,-0.806546515154792));
#16592=CARTESIAN_POINT('',(-5.62,-2.52,0.));
#16593=CARTESIAN_POINT('',(-5.62,0.,0.));
#16594=CARTESIAN_POINT('',(-3.67282446442857,-1.71345348484521,-0.806546515154792));
#16595=CARTESIAN_POINT('Origin',(-2.7,0.,0.));
#16596=CARTESIAN_POINT('',(-2.83,2.52,0.));
#16597=CARTESIAN_POINT('',(-1.35,2.52,0.));
#16598=CARTESIAN_POINT('',(-2.83,-2.52,0.));
#16599=CARTESIAN_POINT('',(-2.83,0.,0.));
#16600=CARTESIAN_POINT('',(-1.35,-2.52,0.));
#16601=CARTESIAN_POINT('Origin',(-1.35,2.56,0.04));
#16602=CARTESIAN_POINT('',(-5.67,2.56464466094067,0.0446446609406727));
#16603=CARTESIAN_POINT('',(-5.67,2.52,0.));
#16604=CARTESIAN_POINT('',(-2.78,2.56464466094067,0.0446446609406727));
#16605=CARTESIAN_POINT('',(-0.675,2.56464466094067,0.0446446609406726));
#16606=CARTESIAN_POINT('',(-2.78,2.54071067811865,0.0207106781186546));
#16607=CARTESIAN_POINT('',(-2.78,2.6,0.0800000000000001));
#16608=CARTESIAN_POINT('',(-2.63667812573082,2.60007654222568,0.0800765422256816));
#16609=CARTESIAN_POINT('Origin',(-5.75,2.52,0.08));
#16610=CARTESIAN_POINT('',(-5.70535533905933,2.56464466094067,0.0800000000000001));
#16611=CARTESIAN_POINT('',(-5.67,2.6,0.0800000000000001));
#16612=CARTESIAN_POINT('',(-5.68306019374819,2.57387961250363,0.0669398062518126));
#16613=CARTESIAN_POINT('',(-6.32870078630161,2.30644652264939,0.445147308951005));
#16614=CARTESIAN_POINT('',(-5.12620462212126,2.18012326166471,-0.883672116214024));
#16615=CARTESIAN_POINT('',(-5.75,2.52,0.08));
#16616=CARTESIAN_POINT('Origin',(-2.78732233047034,0.,0.0176776695296638));
#16617=CARTESIAN_POINT('',(-2.74464466094067,2.52,0.0353553390593276));
#16618=CARTESIAN_POINT('',(-2.29037487135252,2.25389491823563,0.223520046883113));
#16619=CARTESIAN_POINT('',(-2.74464466094067,-2.52,0.0353553390593277));
#16620=CARTESIAN_POINT('',(-2.74464466094067,0.,0.0353553390593275));
#16621=CARTESIAN_POINT('',(-2.78,-2.54071067811865,0.0207106781186546));
#16622=CARTESIAN_POINT('',(-2.25302896331862,-2.23201819180851,0.238989228489893));
#16623=CARTESIAN_POINT('',(-2.63667812573082,-2.60007654222568,0.0800765422256816));
#16624=CARTESIAN_POINT('Origin',(-1.35,-2.56,0.04));
#16625=CARTESIAN_POINT('',(-2.78,-2.56464466094067,0.0446446609406727));
#16626=CARTESIAN_POINT('',(-2.78,-2.52,0.));
#16627=CARTESIAN_POINT('',(-0.675,-2.56464466094067,0.0446446609406726));
#16628=CARTESIAN_POINT('Origin',(-2.7,-2.52,0.0800000000000001));
#16629=CARTESIAN_POINT('',(-2.73535533905933,-2.52,0.0446446609406727));
#16630=CARTESIAN_POINT('',(-2.7,-2.52,0.0800000000000001));
#16631=CARTESIAN_POINT('',(-2.72071067811865,-2.54071067811865,0.0800000000000001));
#16632=CARTESIAN_POINT('',(-2.92352004688311,-2.25389491823563,-0.409625128647479));
#16633=CARTESIAN_POINT('',(-2.74464466094067,-2.56464466094067,0.0800000000000001));
#16634=CARTESIAN_POINT('',(-2.78,-2.6,0.0800000000000001));
#16635=CARTESIAN_POINT('',(-2.76693980625181,-2.57387961250363,0.0669398062518135));
#16636=CARTESIAN_POINT('',(-1.84575441632761,-2.19231213053707,0.606557714209465));
#16637=CARTESIAN_POINT('',(-2.51957511308224,-2.74879286446996,0.489217751387724));
#16638=CARTESIAN_POINT('Origin',(-2.71767766952966,0.,0.087322330470336));
#16639=CARTESIAN_POINT('',(-2.73535533905933,2.52,0.0446446609406726));
#16640=CARTESIAN_POINT('',(-2.73535533905933,0.,0.0446446609406725));
#16641=CARTESIAN_POINT('',(-2.72071067811865,2.54071067811865,0.0800000000000001));
#16642=CARTESIAN_POINT('',(-2.93898922848989,2.23201819180851,-0.44697103668138));
#16643=CARTESIAN_POINT('',(-2.7,2.52,0.129999999999999));
#16644=CARTESIAN_POINT('',(-1.79515397196173,1.61515397196173,2.31449155274942));
#16645=CARTESIAN_POINT('',(-2.7,-2.52,0.129999999999999));
#16646=CARTESIAN_POINT('',(-2.7,0.,0.129999999999999));
#16647=CARTESIAN_POINT('',(-1.79515397196173,-1.61515397196173,2.31449155274942));
#16648=CARTESIAN_POINT('Origin',(-2.7,0.,5.7));
#16649=CARTESIAN_POINT('',(-2.7,2.52,5.36678788880707));
#16650=CARTESIAN_POINT('',(-2.7,2.52,5.0375));
#16651=CARTESIAN_POINT('',(-2.7,2.2,5.3));
#16652=CARTESIAN_POINT('Origin',(-2.7,2.2,6.1));
#16653=CARTESIAN_POINT('',(-2.7,-2.2,5.3));
#16654=CARTESIAN_POINT('',(-2.7,0.,5.3));
#16655=CARTESIAN_POINT('',(-2.7,-2.52,5.36678788880707));
#16656=CARTESIAN_POINT('Origin',(-2.7,-2.2,6.1));
#16657=CARTESIAN_POINT('',(-2.7,-2.52,5.0375));
#16658=CARTESIAN_POINT('',(-2.7,-1.65327317884893E-16,1.65));
#16659=CARTESIAN_POINT('Origin',(-2.7,0.,3.));
#16660=CARTESIAN_POINT('Origin',(-2.74,2.56,5.0375));
#16661=CARTESIAN_POINT('',(-2.74464466094067,2.56464466094067,0.0800000000000001));
#16662=CARTESIAN_POINT('',(-2.7,2.52,0.0800000000000001));
#16663=CARTESIAN_POINT('',(-2.74464466094067,2.56464466094067,5.36678788880707));
#16664=CARTESIAN_POINT('',(-2.74464466094067,2.56464466094067,4.70625));
#16665=CARTESIAN_POINT('',(-2.78,2.6,5.36678788880707));
#16666=CARTESIAN_POINT('Origin',(-2.78,2.52,0.));
#16667=CARTESIAN_POINT('',(-2.76693980625181,2.57387961250363,0.0669398062518129));
#16668=CARTESIAN_POINT('',(-2.54410593147546,2.73144695643606,0.447341024960603));
#16669=CARTESIAN_POINT('',(-1.88763114275473,2.20965803857097,0.582026895816245));
#16670=CARTESIAN_POINT('',(-2.78,2.52,0.));
#16671=CARTESIAN_POINT('Origin',(-0.675,-2.58232233047034,0.0873223304703362));
#16672=CARTESIAN_POINT('',(-2.83,-2.6,0.13));
#16673=CARTESIAN_POINT('',(-3.36446283715638,-2.82138175573458,0.664462837156383));
#16674=CARTESIAN_POINT('',(-5.62,-2.6,0.13));
#16675=CARTESIAN_POINT('',(-0.675,-2.6,0.13));
#16676=CARTESIAN_POINT('',(-3.77888057658085,-3.36261663512876,1.97111942341917));
#16677=CARTESIAN_POINT('Origin',(-2.78732233047034,-2.58232233047034,4.70625));
#16678=CARTESIAN_POINT('',(-2.74464466094067,-2.56464466094067,5.36678788880707));
#16679=CARTESIAN_POINT('',(-2.74464466094067,-2.56464466094067,4.70625));
#16680=CARTESIAN_POINT('',(-2.83,-2.6,5.36678788880707));
#16681=CARTESIAN_POINT('',(-2.83,-2.6,5.36678788880707));
#16682=CARTESIAN_POINT('',(-2.83,-2.6,4.70625));
#16683=CARTESIAN_POINT('Ctrl Pts',(-2.74442178368363,-2.56486895213994,
5.39792313687514));
#16684=CARTESIAN_POINT('Ctrl Pts',(-2.74456950540178,-2.56471935013366,
5.38754472085245));
#16685=CARTESIAN_POINT('Ctrl Pts',(-2.74464466094067,-2.56464466094067,
5.37716630482976));
#16686=CARTESIAN_POINT('Ctrl Pts',(-2.74464466094067,-2.56464466094067,
5.36678788880707));
#16687=CARTESIAN_POINT('Ctrl Pts',(-2.77294785578909,-2.57657930142663,
5.39792313687514));
#16688=CARTESIAN_POINT('Ctrl Pts',(-2.77304633693452,-2.57647956675577,
5.38754472085245));
#16689=CARTESIAN_POINT('Ctrl Pts',(-2.77309644062712,-2.57642977396045,
5.37716630482976));
#16690=CARTESIAN_POINT('Ctrl Pts',(-2.77309644062712,-2.57642977396045,
5.36678788880707));
#16691=CARTESIAN_POINT('Ctrl Pts',(-2.80147392789454,-2.58828965071331,
5.39792313687514));
#16692=CARTESIAN_POINT('Ctrl Pts',(-2.80152316846726,-2.58823978337789,
5.38754472085245));
#16693=CARTESIAN_POINT('Ctrl Pts',(-2.80154822031356,-2.58821488698022,
5.37716630482976));
#16694=CARTESIAN_POINT('Ctrl Pts',(-2.80154822031356,-2.58821488698022,
5.36678788880707));
#16695=CARTESIAN_POINT('Ctrl Pts',(-2.83,-2.6,5.39792313687514));
#16696=CARTESIAN_POINT('Ctrl Pts',(-2.83,-2.6,5.38754472085245));
#16697=CARTESIAN_POINT('Ctrl Pts',(-2.83,-2.6,5.37716630482976));
#16698=CARTESIAN_POINT('Ctrl Pts',(-2.83,-2.6,5.36678788880707));
#16699=CARTESIAN_POINT('',(-2.74442178368363,-2.56486895213994,5.39792313687514));
#16700=CARTESIAN_POINT('',(-2.83,-2.6,5.39792313687514));
#16701=CARTESIAN_POINT('Ctrl Pts',(-2.74442178368363,-2.56486895213994,
5.39792313687514));
#16702=CARTESIAN_POINT('Ctrl Pts',(-2.77294785578909,-2.57657930142663,
5.39792313687514));
#16703=CARTESIAN_POINT('Ctrl Pts',(-2.80147392789454,-2.58828965071331,
5.39792313687514));
#16704=CARTESIAN_POINT('Ctrl Pts',(-2.83,-2.6,5.39792313687514));
#16705=CARTESIAN_POINT('Ctrl Pts',(-2.83,-2.6,5.39792313687514));
#16706=CARTESIAN_POINT('Ctrl Pts',(-2.83,-2.6,5.38754472085245));
#16707=CARTESIAN_POINT('Ctrl Pts',(-2.83,-2.6,5.37716630482976));
#16708=CARTESIAN_POINT('Ctrl Pts',(-2.83,-2.6,5.36678788880707));
#16709=CARTESIAN_POINT('Ctrl Pts',(-2.74464466094067,-2.56464466094067,
5.36678788880707));
#16710=CARTESIAN_POINT('Ctrl Pts',(-2.74464466094067,-2.56464466094067,
5.37716630482976));
#16711=CARTESIAN_POINT('Ctrl Pts',(-2.74456950540178,-2.56471935013366,
5.38754472085245));
#16712=CARTESIAN_POINT('Ctrl Pts',(-2.74442178368363,-2.56486895213994,
5.39792313687514));
#16713=CARTESIAN_POINT('Ctrl Pts',(-2.74442178368363,-2.56486895213994,
5.39792313687514));
#16714=CARTESIAN_POINT('Ctrl Pts',(-2.75619335349611,-2.57658041242369,
5.40100865024091));
#16715=CARTESIAN_POINT('Ctrl Pts',(-2.76803982089572,-2.58829135908796,
5.40409416360668));
#16716=CARTESIAN_POINT('Ctrl Pts',(-2.78,-2.6,5.40717967697245));
#16717=CARTESIAN_POINT('Ctrl Pts',(-2.77294785578909,-2.57657930142663,
5.39792313687514));
#16718=CARTESIAN_POINT('Ctrl Pts',(-2.77524001344185,-2.58438694161579,
5.40100865024091));
#16719=CARTESIAN_POINT('Ctrl Pts',(-2.77758210281937,-2.59219423939197,
5.40409416360668));
#16720=CARTESIAN_POINT('Ctrl Pts',(-2.78,-2.6,5.40717967697245));
#16721=CARTESIAN_POINT('Ctrl Pts',(-2.80147392789454,-2.58828965071331,
5.39792313687514));
#16722=CARTESIAN_POINT('Ctrl Pts',(-2.79428667338759,-2.5921934708079,5.40100865024091));
#16723=CARTESIAN_POINT('Ctrl Pts',(-2.78712438474302,-2.59609711969599,
5.40409416360668));
#16724=CARTESIAN_POINT('Ctrl Pts',(-2.78,-2.6,5.40717967697245));
#16725=CARTESIAN_POINT('Ctrl Pts',(-2.83,-2.6,5.39792313687514));
#16726=CARTESIAN_POINT('Ctrl Pts',(-2.81333333333333,-2.6,5.40100865024091));
#16727=CARTESIAN_POINT('Ctrl Pts',(-2.79666666666667,-2.6,5.40409416360668));
#16728=CARTESIAN_POINT('Ctrl Pts',(-2.78,-2.6,5.40717967697245));
#16729=CARTESIAN_POINT('',(-2.78,-2.6,5.40717967697245));
#16730=CARTESIAN_POINT('Ctrl Pts',(-2.74442178368363,-2.56486895213994,
5.39792313687514));
#16731=CARTESIAN_POINT('Ctrl Pts',(-2.75619335349611,-2.57658041242369,
5.40100865024091));
#16732=CARTESIAN_POINT('Ctrl Pts',(-2.76803982089572,-2.58829135908796,
5.40409416360668));
#16733=CARTESIAN_POINT('Ctrl Pts',(-2.78,-2.6,5.40717967697245));
#16734=CARTESIAN_POINT('Ctrl Pts',(-2.78,-2.6,5.40717967697245));
#16735=CARTESIAN_POINT('Ctrl Pts',(-2.79666666666667,-2.6,5.40409416360668));
#16736=CARTESIAN_POINT('Ctrl Pts',(-2.81333333333333,-2.6,5.40100865024091));
#16737=CARTESIAN_POINT('Ctrl Pts',(-2.83,-2.6,5.39792313687514));
#16738=CARTESIAN_POINT('Origin',(0.,-2.6,4.375));
#16739=CARTESIAN_POINT('',(-2.42414283215669,-2.6,6.08851340213307));
#16740=CARTESIAN_POINT('Ctrl Pts',(-2.42414283215669,-2.6,6.08851340213307));
#16741=CARTESIAN_POINT('Ctrl Pts',(-2.47340183676932,-2.6,6.03819996865104));
#16742=CARTESIAN_POINT('Ctrl Pts',(-2.55014714354309,-2.6,5.9563590107329));
#16743=CARTESIAN_POINT('Ctrl Pts',(-2.6396310734963,-2.6,5.83483846916786));
#16744=CARTESIAN_POINT('Ctrl Pts',(-2.69414240597218,-2.6,5.74352625586477));
#16745=CARTESIAN_POINT('Ctrl Pts',(-2.74081734015966,-2.6,5.6395635803662));
#16746=CARTESIAN_POINT('Ctrl Pts',(-2.77299866241655,-2.6,5.52278122462383));
#16747=CARTESIAN_POINT('Ctrl Pts',(-2.78,-2.6,5.44464477671195));
#16748=CARTESIAN_POINT('Ctrl Pts',(-2.78,-2.6,5.40717967697245));
#16749=CARTESIAN_POINT('',(-2.3,-2.6,6.1));
#16750=CARTESIAN_POINT('Ctrl Pts',(-2.3,-2.6,6.1));
#16751=CARTESIAN_POINT('Ctrl Pts',(-2.34138094405223,-2.6,6.09617113404436));
#16752=CARTESIAN_POINT('Ctrl Pts',(-2.38276188810446,-2.6,6.09234226808871));
#16753=CARTESIAN_POINT('Ctrl Pts',(-2.42414283215669,-2.6,6.08851340213307));
#16754=CARTESIAN_POINT('',(2.3,-2.6,6.1));
#16755=CARTESIAN_POINT('',(1.35,-2.6,6.1));
#16756=CARTESIAN_POINT('',(2.42414283239008,-2.6,6.08851340189468));
#16757=CARTESIAN_POINT('Ctrl Pts',(2.42414283239008,-2.6,6.08851340189468));
#16758=CARTESIAN_POINT('Ctrl Pts',(2.38276188826005,-2.6,6.09234226792978));
#16759=CARTESIAN_POINT('Ctrl Pts',(2.34138094413003,-2.6,6.09617113396489));
#16760=CARTESIAN_POINT('Ctrl Pts',(2.3,-2.6,6.1));
#16761=CARTESIAN_POINT('',(2.78,-2.6,5.40717967697245));
#16762=CARTESIAN_POINT('Ctrl Pts',(2.78,-2.6,5.40717967697245));
#16763=CARTESIAN_POINT('Ctrl Pts',(2.78,-2.6,5.44865469871872));
#16764=CARTESIAN_POINT('Ctrl Pts',(2.77175013108469,-2.6,5.53495446115542));
#16765=CARTESIAN_POINT('Ctrl Pts',(2.73152937534889,-2.6,5.66466680090526));
#16766=CARTESIAN_POINT('Ctrl Pts',(2.66093134122623,-2.6,5.80894311125375));
#16767=CARTESIAN_POINT('Ctrl Pts',(2.5873706385557,-2.6,5.90812597923557));
#16768=CARTESIAN_POINT('Ctrl Pts',(2.49738496881261,-2.6,6.0124608445315));
#16769=CARTESIAN_POINT('Ctrl Pts',(2.46022125233207,-2.6,6.05166269416259));
#16770=CARTESIAN_POINT('Ctrl Pts',(2.42414283239008,-2.6,6.08851340189468));
#16771=CARTESIAN_POINT('',(2.83,-2.6,5.39792313665174));
#16772=CARTESIAN_POINT('Ctrl Pts',(2.83,-2.6,5.39792313665174));
#16773=CARTESIAN_POINT('Ctrl Pts',(2.81333333333333,-2.6,5.40100865009198));
#16774=CARTESIAN_POINT('Ctrl Pts',(2.79666666666667,-2.6,5.40409416353221));
#16775=CARTESIAN_POINT('Ctrl Pts',(2.78,-2.6,5.40717967697245));
#16776=CARTESIAN_POINT('',(2.83,-2.6,5.36678788880707));
#16777=CARTESIAN_POINT('Ctrl Pts',(2.83,-2.6,5.36678788880707));
#16778=CARTESIAN_POINT('Ctrl Pts',(2.83,-2.6,5.37716630475529));
#16779=CARTESIAN_POINT('Ctrl Pts',(2.83,-2.6,5.38754472070352));
#16780=CARTESIAN_POINT('Ctrl Pts',(2.83,-2.6,5.39792313665175));
#16781=CARTESIAN_POINT('',(2.83,-2.6,0.13));
#16782=CARTESIAN_POINT('',(2.83,-2.6,3.28125));
#16783=CARTESIAN_POINT('',(5.62,-2.6,0.13));
#16784=CARTESIAN_POINT('',(1.4375,-2.6,0.13));
#16785=CARTESIAN_POINT('',(5.62,-2.6,8.62));
#16786=CARTESIAN_POINT('',(5.62,-2.6,5.46875));
#16787=CARTESIAN_POINT('',(-5.62,-2.6,8.62));
#16788=CARTESIAN_POINT('',(-1.4375,-2.6,8.62));
#16789=CARTESIAN_POINT('',(-5.62,-2.6,3.28125));
#16790=CARTESIAN_POINT('',(4.21,-2.6,1.));
#16791=CARTESIAN_POINT('Origin',(4.6,-2.6,1.));
#16792=CARTESIAN_POINT('',(-4.99,-2.6,1.));
#16793=CARTESIAN_POINT('Origin',(-4.6,-2.6,1.));
#16794=CARTESIAN_POINT('',(4.21,-2.6,7.75));
#16795=CARTESIAN_POINT('Origin',(4.6,-2.6,7.75));
#16796=CARTESIAN_POINT('',(-4.99,-2.6,7.75));
#16797=CARTESIAN_POINT('Origin',(-4.6,-2.6,7.75));
#16798=CARTESIAN_POINT('Ctrl Pts',(-2.69829980684391,-2.52001806864527,
5.40717967697245));
#16799=CARTESIAN_POINT('Ctrl Pts',(-2.69942945076934,-2.51999405556084,
5.39371574758399));
#16800=CARTESIAN_POINT('Ctrl Pts',(-2.7,-2.52,5.38025181819553));
#16801=CARTESIAN_POINT('Ctrl Pts',(-2.7,-2.52,5.36678788880707));
#16802=CARTESIAN_POINT('Ctrl Pts',(-2.7255332045626,-2.54667871243018,5.40717967697245));
#16803=CARTESIAN_POINT('Ctrl Pts',(-2.72628630051289,-2.54666270370723,
5.39371574758399));
#16804=CARTESIAN_POINT('Ctrl Pts',(-2.72666666666667,-2.54666666666667,
5.38025181819553));
#16805=CARTESIAN_POINT('Ctrl Pts',(-2.72666666666667,-2.54666666666667,
5.36678788880707));
#16806=CARTESIAN_POINT('Ctrl Pts',(-2.7527666022813,-2.57333935621509,5.40717967697245));
#16807=CARTESIAN_POINT('Ctrl Pts',(-2.75314315025645,-2.57333135185361,
5.39371574758399));
#16808=CARTESIAN_POINT('Ctrl Pts',(-2.75333333333333,-2.57333333333333,
5.38025181819553));
#16809=CARTESIAN_POINT('Ctrl Pts',(-2.75333333333333,-2.57333333333333,
5.36678788880707));
#16810=CARTESIAN_POINT('Ctrl Pts',(-2.78,-2.6,5.40717967697245));
#16811=CARTESIAN_POINT('Ctrl Pts',(-2.78,-2.6,5.39371574758399));
#16812=CARTESIAN_POINT('Ctrl Pts',(-2.78,-2.6,5.38025181819553));
#16813=CARTESIAN_POINT('Ctrl Pts',(-2.78,-2.6,5.36678788880707));
#16814=CARTESIAN_POINT('',(-2.7,-2.52,5.36678788880707));
#16815=CARTESIAN_POINT('',(-2.69829980684391,-2.52001806864527,5.40717967697245));
#16816=CARTESIAN_POINT('Ctrl Pts',(-2.7,-2.52,5.36678788880707));
#16817=CARTESIAN_POINT('Ctrl Pts',(-2.7,-2.52,5.38025181819553));
#16818=CARTESIAN_POINT('Ctrl Pts',(-2.69942945076934,-2.51999405556084,
5.39371574758399));
#16819=CARTESIAN_POINT('Ctrl Pts',(-2.69829980684391,-2.52001806864527,
5.40717967697245));
#16820=CARTESIAN_POINT('',(-2.78,-2.6,5.40717967697245));
#16821=CARTESIAN_POINT('Origin',(-1.4375,-2.58232233047034,8.66267766952966));
#16822=CARTESIAN_POINT('',(-3.45077738091134,-3.49852142863302,6.45077738091131));
#16823=CARTESIAN_POINT('',(3.29248197949184,-3.56408953076227,6.29248197949182));
#16824=CARTESIAN_POINT('Origin',(-5.66267766952966,-2.58232233047034,3.28125));
#16825=CARTESIAN_POINT('Origin',(1.4375,-2.58232233047034,0.0873223304703362));
#16826=CARTESIAN_POINT('',(3.45077738091134,-3.49852142863302,2.29922261908869));
#16827=CARTESIAN_POINT('',(3.21192363215214,-2.75819794822821,0.511923632152139));
#16828=CARTESIAN_POINT('Origin',(5.66267766952966,-2.58232233047034,5.46875));
#16829=CARTESIAN_POINT('Origin',(2.78732233047034,-2.58232233047034,3.28125));
#16830=CARTESIAN_POINT('',(2.83,-2.6,5.36678788880707));
#16831=CARTESIAN_POINT('Ctrl Pts',(2.74464466094067,-2.56464466094067,5.36678788880707));
#16832=CARTESIAN_POINT('Ctrl Pts',(2.74464466094067,-2.56464466094067,5.37716630475529));
#16833=CARTESIAN_POINT('Ctrl Pts',(2.74456950540286,-2.56471935013259,5.38754472070352));
#16834=CARTESIAN_POINT('Ctrl Pts',(2.74442178368681,-2.56486895213672,5.39792313665175));
#16835=CARTESIAN_POINT('Ctrl Pts',(2.77309644062712,-2.57642977396045,5.36678788880707));
#16836=CARTESIAN_POINT('Ctrl Pts',(2.77309644062712,-2.57642977396045,5.37716630475529));
#16837=CARTESIAN_POINT('Ctrl Pts',(2.77304633693524,-2.57647956675506,5.38754472070352));
#16838=CARTESIAN_POINT('Ctrl Pts',(2.77294785579121,-2.57657930142448,5.39792313665175));
#16839=CARTESIAN_POINT('Ctrl Pts',(2.80154822031356,-2.58821488698022,5.36678788880707));
#16840=CARTESIAN_POINT('Ctrl Pts',(2.80154822031356,-2.58821488698022,5.37716630475529));
#16841=CARTESIAN_POINT('Ctrl Pts',(2.80152316846762,-2.58823978337753,5.38754472070352));
#16842=CARTESIAN_POINT('Ctrl Pts',(2.8014739278956,-2.58828965071224,5.39792313665175));
#16843=CARTESIAN_POINT('Ctrl Pts',(2.83,-2.6,5.36678788880707));
#16844=CARTESIAN_POINT('Ctrl Pts',(2.83,-2.6,5.37716630475529));
#16845=CARTESIAN_POINT('Ctrl Pts',(2.83,-2.6,5.38754472070352));
#16846=CARTESIAN_POINT('Ctrl Pts',(2.83,-2.6,5.39792313665175));
#16847=CARTESIAN_POINT('',(2.74442178368681,-2.56486895213672,5.39792313665174));
#16848=CARTESIAN_POINT('Ctrl Pts',(2.83,-2.6,5.39792313665175));
#16849=CARTESIAN_POINT('Ctrl Pts',(2.8014739278956,-2.58828965071224,5.39792313665175));
#16850=CARTESIAN_POINT('Ctrl Pts',(2.77294785579121,-2.57657930142448,5.39792313665175));
#16851=CARTESIAN_POINT('Ctrl Pts',(2.74442178368681,-2.56486895213672,5.39792313665175));
#16852=CARTESIAN_POINT('Ctrl Pts',(2.74442178368681,-2.56486895213672,5.39792313665175));
#16853=CARTESIAN_POINT('Ctrl Pts',(2.74456950540286,-2.56471935013259,5.38754472070352));
#16854=CARTESIAN_POINT('Ctrl Pts',(2.74464466094067,-2.56464466094067,5.37716630475529));
#16855=CARTESIAN_POINT('Ctrl Pts',(2.74464466094067,-2.56464466094067,5.36678788880707));
#16856=CARTESIAN_POINT('Ctrl Pts',(2.83,-2.6,5.39792313665174));
#16857=CARTESIAN_POINT('Ctrl Pts',(2.81333333333333,-2.6,5.40100865009198));
#16858=CARTESIAN_POINT('Ctrl Pts',(2.79666666666667,-2.6,5.40409416353221));
#16859=CARTESIAN_POINT('Ctrl Pts',(2.78,-2.6,5.40717967697245));
#16860=CARTESIAN_POINT('Ctrl Pts',(2.8014739278956,-2.58828965071224,5.39792313665174));
#16861=CARTESIAN_POINT('Ctrl Pts',(2.7942866733878,-2.59219347080718,5.40100865009198));
#16862=CARTESIAN_POINT('Ctrl Pts',(2.78712438474266,-2.59609711969564,5.40409416353221));
#16863=CARTESIAN_POINT('Ctrl Pts',(2.78,-2.6,5.40717967697245));
#16864=CARTESIAN_POINT('Ctrl Pts',(2.77294785579121,-2.57657930142448,5.39792313665174));
#16865=CARTESIAN_POINT('Ctrl Pts',(2.77524001344226,-2.58438694161436,5.40100865009198));
#16866=CARTESIAN_POINT('Ctrl Pts',(2.77758210281866,-2.59219423939128,5.40409416353221));
#16867=CARTESIAN_POINT('Ctrl Pts',(2.78,-2.6,5.40717967697245));
#16868=CARTESIAN_POINT('Ctrl Pts',(2.74442178368681,-2.56486895213672,5.39792313665174));
#16869=CARTESIAN_POINT('Ctrl Pts',(2.75619335349672,-2.57658041242155,5.40100865009198));
#16870=CARTESIAN_POINT('Ctrl Pts',(2.76803982089465,-2.58829135908692,5.40409416353221));
#16871=CARTESIAN_POINT('Ctrl Pts',(2.78,-2.6,5.40717967697245));
#16872=CARTESIAN_POINT('Ctrl Pts',(2.78,-2.6,5.40717967697245));
#16873=CARTESIAN_POINT('Ctrl Pts',(2.76803982089465,-2.58829135908692,5.40409416353221));
#16874=CARTESIAN_POINT('Ctrl Pts',(2.75619335349672,-2.57658041242155,5.40100865009198));
#16875=CARTESIAN_POINT('Ctrl Pts',(2.74442178368681,-2.56486895213672,5.39792313665174));
#16876=CARTESIAN_POINT('Origin',(1.4375,2.58232233047034,0.0873223304703362));
#16877=CARTESIAN_POINT('',(2.83,2.6,0.13));
#16878=CARTESIAN_POINT('',(3.21192363215214,2.75819794822821,0.511923632152139));
#16879=CARTESIAN_POINT('',(5.62,2.6,0.13));
#16880=CARTESIAN_POINT('',(1.4375,2.6,0.13));
#16881=CARTESIAN_POINT('',(3.45077738091134,3.49852142863302,2.29922261908869));
#16882=CARTESIAN_POINT('Origin',(2.78732233047034,2.58232233047034,3.28125));
#16883=CARTESIAN_POINT('',(2.74464466094067,2.56464466094067,5.36678788880707));
#16884=CARTESIAN_POINT('',(2.74464466094067,2.56464466094067,3.28125));
#16885=CARTESIAN_POINT('',(2.83,2.6,5.36678788880707));
#16886=CARTESIAN_POINT('',(2.83,2.6,5.36678788880707));
#16887=CARTESIAN_POINT('',(2.83,2.6,3.28125));
#16888=CARTESIAN_POINT('Ctrl Pts',(2.74442178368363,2.56486895213994,5.39792313687514));
#16889=CARTESIAN_POINT('Ctrl Pts',(2.74456950540177,2.56471935013366,5.38754472085245));
#16890=CARTESIAN_POINT('Ctrl Pts',(2.74464466094067,2.56464466094067,5.37716630482976));
#16891=CARTESIAN_POINT('Ctrl Pts',(2.74464466094067,2.56464466094067,5.36678788880707));
#16892=CARTESIAN_POINT('Ctrl Pts',(2.77294785578909,2.57657930142663,5.39792313687514));
#16893=CARTESIAN_POINT('Ctrl Pts',(2.77304633693452,2.57647956675577,5.38754472085245));
#16894=CARTESIAN_POINT('Ctrl Pts',(2.77309644062712,2.57642977396045,5.37716630482976));
#16895=CARTESIAN_POINT('Ctrl Pts',(2.77309644062712,2.57642977396045,5.36678788880707));
#16896=CARTESIAN_POINT('Ctrl Pts',(2.80147392789454,2.58828965071331,5.39792313687514));
#16897=CARTESIAN_POINT('Ctrl Pts',(2.80152316846726,2.58823978337789,5.38754472085245));
#16898=CARTESIAN_POINT('Ctrl Pts',(2.80154822031356,2.58821488698022,5.37716630482976));
#16899=CARTESIAN_POINT('Ctrl Pts',(2.80154822031356,2.58821488698022,5.36678788880707));
#16900=CARTESIAN_POINT('Ctrl Pts',(2.83,2.6,5.39792313687514));
#16901=CARTESIAN_POINT('Ctrl Pts',(2.83,2.6,5.38754472085245));
#16902=CARTESIAN_POINT('Ctrl Pts',(2.83,2.6,5.37716630482976));
#16903=CARTESIAN_POINT('Ctrl Pts',(2.83,2.6,5.36678788880707));
#16904=CARTESIAN_POINT('',(2.74442178368363,2.56486895213994,5.39792313687514));
#16905=CARTESIAN_POINT('',(2.83,2.6,5.39792313687514));
#16906=CARTESIAN_POINT('Ctrl Pts',(2.74442178368363,2.56486895213994,5.39792313687514));
#16907=CARTESIAN_POINT('Ctrl Pts',(2.77294785578909,2.57657930142663,5.39792313687514));
#16908=CARTESIAN_POINT('Ctrl Pts',(2.80147392789454,2.58828965071331,5.39792313687514));
#16909=CARTESIAN_POINT('Ctrl Pts',(2.83,2.6,5.39792313687514));
#16910=CARTESIAN_POINT('Ctrl Pts',(2.83,2.6,5.39792313687514));
#16911=CARTESIAN_POINT('Ctrl Pts',(2.83,2.6,5.38754472085245));
#16912=CARTESIAN_POINT('Ctrl Pts',(2.83,2.6,5.37716630482976));
#16913=CARTESIAN_POINT('Ctrl Pts',(2.83,2.6,5.36678788880707));
#16914=CARTESIAN_POINT('Ctrl Pts',(2.74464466094067,2.56464466094067,5.36678788880707));
#16915=CARTESIAN_POINT('Ctrl Pts',(2.74464466094067,2.56464466094067,5.37716630482976));
#16916=CARTESIAN_POINT('Ctrl Pts',(2.74456950540177,2.56471935013366,5.38754472085245));
#16917=CARTESIAN_POINT('Ctrl Pts',(2.74442178368363,2.56486895213994,5.39792313687514));
#16918=CARTESIAN_POINT('Ctrl Pts',(2.74442178368363,2.56486895213994,5.39792313687514));
#16919=CARTESIAN_POINT('Ctrl Pts',(2.75619335349611,2.57658041242369,5.40100865024091));
#16920=CARTESIAN_POINT('Ctrl Pts',(2.76803982089572,2.58829135908796,5.40409416360668));
#16921=CARTESIAN_POINT('Ctrl Pts',(2.78,2.6,5.40717967697245));
#16922=CARTESIAN_POINT('Ctrl Pts',(2.77294785578909,2.57657930142663,5.39792313687514));
#16923=CARTESIAN_POINT('Ctrl Pts',(2.77524001344185,2.58438694161579,5.40100865024091));
#16924=CARTESIAN_POINT('Ctrl Pts',(2.77758210281937,2.59219423939197,5.40409416360668));
#16925=CARTESIAN_POINT('Ctrl Pts',(2.78,2.6,5.40717967697245));
#16926=CARTESIAN_POINT('Ctrl Pts',(2.80147392789454,2.58828965071331,5.39792313687514));
#16927=CARTESIAN_POINT('Ctrl Pts',(2.79428667338759,2.5921934708079,5.40100865024091));
#16928=CARTESIAN_POINT('Ctrl Pts',(2.78712438474302,2.59609711969599,5.40409416360668));
#16929=CARTESIAN_POINT('Ctrl Pts',(2.78,2.6,5.40717967697245));
#16930=CARTESIAN_POINT('Ctrl Pts',(2.83,2.6,5.39792313687514));
#16931=CARTESIAN_POINT('Ctrl Pts',(2.81333333333333,2.6,5.40100865024091));
#16932=CARTESIAN_POINT('Ctrl Pts',(2.79666666666667,2.6,5.40409416360668));
#16933=CARTESIAN_POINT('Ctrl Pts',(2.78,2.6,5.40717967697245));
#16934=CARTESIAN_POINT('',(2.78,2.6,5.40717967697245));
#16935=CARTESIAN_POINT('Ctrl Pts',(2.74442178368363,2.56486895213994,5.39792313687514));
#16936=CARTESIAN_POINT('Ctrl Pts',(2.75619335349611,2.57658041242369,5.40100865024091));
#16937=CARTESIAN_POINT('Ctrl Pts',(2.76803982089572,2.58829135908796,5.40409416360668));
#16938=CARTESIAN_POINT('Ctrl Pts',(2.78,2.6,5.40717967697245));
#16939=CARTESIAN_POINT('Ctrl Pts',(2.78,2.6,5.40717967697245));
#16940=CARTESIAN_POINT('Ctrl Pts',(2.79666666666667,2.6,5.40409416360668));
#16941=CARTESIAN_POINT('Ctrl Pts',(2.81333333333333,2.6,5.40100865024091));
#16942=CARTESIAN_POINT('Ctrl Pts',(2.83,2.6,5.39792313687514));
#16943=CARTESIAN_POINT('Origin',(0.,2.6,4.375));
#16944=CARTESIAN_POINT('',(2.42414283215735,2.6,6.0885134021324));
#16945=CARTESIAN_POINT('Ctrl Pts',(2.42414283215735,2.6,6.0885134021324));
#16946=CARTESIAN_POINT('Ctrl Pts',(2.47340183676993,2.6,6.03819996865039));
#16947=CARTESIAN_POINT('Ctrl Pts',(2.57677270784915,2.6,5.92754153415384));
#16948=CARTESIAN_POINT('Ctrl Pts',(2.66963073857957,2.6,5.79083331222164));
#16949=CARTESIAN_POINT('Ctrl Pts',(2.7334746318431,2.6,5.65860602138498));
#16950=CARTESIAN_POINT('Ctrl Pts',(2.77172491031876,2.6,5.54191130109615));
#16951=CARTESIAN_POINT('Ctrl Pts',(2.78,2.6,5.44464477671191));
#16952=CARTESIAN_POINT('Ctrl Pts',(2.78,2.6,5.40717967697245));
#16953=CARTESIAN_POINT('',(2.3,2.6,6.1));
#16954=CARTESIAN_POINT('Ctrl Pts',(2.3,2.6,6.1));
#16955=CARTESIAN_POINT('Ctrl Pts',(2.34138094405245,2.6,6.09617113404413));
#16956=CARTESIAN_POINT('Ctrl Pts',(2.3827618881049,2.6,6.09234226808826));
#16957=CARTESIAN_POINT('Ctrl Pts',(2.42414283215735,2.6,6.0885134021324));
#16958=CARTESIAN_POINT('',(-2.3,2.6,6.1));
#16959=CARTESIAN_POINT('',(1.35,2.6,6.1));
#16960=CARTESIAN_POINT('',(-2.42414283238944,2.6,6.08851340189533));
#16961=CARTESIAN_POINT('Ctrl Pts',(-2.42414283238944,2.6,6.08851340189533));
#16962=CARTESIAN_POINT('Ctrl Pts',(-2.38276188825963,2.6,6.09234226793022));
#16963=CARTESIAN_POINT('Ctrl Pts',(-2.34138094412981,2.6,6.09617113396511));
#16964=CARTESIAN_POINT('Ctrl Pts',(-2.3,2.6,6.1));
#16965=CARTESIAN_POINT('',(-2.78,2.6,5.40717967697245));
#16966=CARTESIAN_POINT('Ctrl Pts',(-2.78,2.6,5.40717967697245));
#16967=CARTESIAN_POINT('Ctrl Pts',(-2.78,2.6,5.44865469871872));
#16968=CARTESIAN_POINT('Ctrl Pts',(-2.77175013108469,2.6,5.53495446115542));
#16969=CARTESIAN_POINT('Ctrl Pts',(-2.7315293753489,2.6,5.66466680090526));
#16970=CARTESIAN_POINT('Ctrl Pts',(-2.66093134122624,2.6,5.80894311125375));
#16971=CARTESIAN_POINT('Ctrl Pts',(-2.5873706385557,2.6,5.90812597923557));
#16972=CARTESIAN_POINT('Ctrl Pts',(-2.4973849688124,2.6,6.01246084453175));
#16973=CARTESIAN_POINT('Ctrl Pts',(-2.46022125233163,2.6,6.05166269416306));
#16974=CARTESIAN_POINT('Ctrl Pts',(-2.42414283238944,2.6,6.08851340189533));
#16975=CARTESIAN_POINT('',(-2.83,2.6,5.39792313665175));
#16976=CARTESIAN_POINT('Ctrl Pts',(-2.83,2.6,5.39792313665175));
#16977=CARTESIAN_POINT('Ctrl Pts',(-2.81333333333333,2.6,5.40100865009198));
#16978=CARTESIAN_POINT('Ctrl Pts',(-2.79666666666667,2.6,5.40409416353221));
#16979=CARTESIAN_POINT('Ctrl Pts',(-2.78,2.6,5.40717967697245));
#16980=CARTESIAN_POINT('',(-2.83,2.6,5.36678788880707));
#16981=CARTESIAN_POINT('Ctrl Pts',(-2.83,2.6,5.36678788880707));
#16982=CARTESIAN_POINT('Ctrl Pts',(-2.83,2.6,5.37716630475529));
#16983=CARTESIAN_POINT('Ctrl Pts',(-2.83,2.6,5.38754472070352));
#16984=CARTESIAN_POINT('Ctrl Pts',(-2.83,2.6,5.39792313665175));
#16985=CARTESIAN_POINT('',(-2.83,2.6,0.13));
#16986=CARTESIAN_POINT('',(-2.83,2.6,4.70625));
#16987=CARTESIAN_POINT('',(-5.62,2.6,0.13));
#16988=CARTESIAN_POINT('',(-0.675,2.6,0.13));
#16989=CARTESIAN_POINT('',(-5.62,2.6,8.62));
#16990=CARTESIAN_POINT('',(-5.62,2.6,3.28125));
#16991=CARTESIAN_POINT('',(5.62,2.6,8.62));
#16992=CARTESIAN_POINT('',(-1.4375,2.6,8.62));
#16993=CARTESIAN_POINT('',(5.62,2.6,5.46875));
#16994=CARTESIAN_POINT('',(4.21,2.6,1.));
#16995=CARTESIAN_POINT('Origin',(4.6,2.6,1.));
#16996=CARTESIAN_POINT('',(-4.99,2.6,1.));
#16997=CARTESIAN_POINT('Origin',(-4.6,2.6,1.));
#16998=CARTESIAN_POINT('',(4.21,2.6,7.75));
#16999=CARTESIAN_POINT('Origin',(4.6,2.6,7.75));
#17000=CARTESIAN_POINT('',(-4.99,2.6,7.75));
#17001=CARTESIAN_POINT('Origin',(-4.6,2.6,7.75));
#17002=CARTESIAN_POINT('Ctrl Pts',(2.69829980684391,2.52001806864527,5.40717967697245));
#17003=CARTESIAN_POINT('Ctrl Pts',(2.69942945076934,2.51999405556084,5.39371574758399));
#17004=CARTESIAN_POINT('Ctrl Pts',(2.7,2.52,5.38025181819553));
#17005=CARTESIAN_POINT('Ctrl Pts',(2.7,2.52,5.36678788880707));
#17006=CARTESIAN_POINT('Ctrl Pts',(2.7255332045626,2.54667871243018,5.40717967697245));
#17007=CARTESIAN_POINT('Ctrl Pts',(2.72628630051289,2.54666270370723,5.39371574758399));
#17008=CARTESIAN_POINT('Ctrl Pts',(2.72666666666667,2.54666666666667,5.38025181819553));
#17009=CARTESIAN_POINT('Ctrl Pts',(2.72666666666667,2.54666666666667,5.36678788880707));
#17010=CARTESIAN_POINT('Ctrl Pts',(2.7527666022813,2.57333935621509,5.40717967697245));
#17011=CARTESIAN_POINT('Ctrl Pts',(2.75314315025645,2.57333135185361,5.39371574758399));
#17012=CARTESIAN_POINT('Ctrl Pts',(2.75333333333333,2.57333333333333,5.38025181819553));
#17013=CARTESIAN_POINT('Ctrl Pts',(2.75333333333333,2.57333333333333,5.36678788880707));
#17014=CARTESIAN_POINT('Ctrl Pts',(2.78,2.6,5.40717967697245));
#17015=CARTESIAN_POINT('Ctrl Pts',(2.78,2.6,5.39371574758399));
#17016=CARTESIAN_POINT('Ctrl Pts',(2.78,2.6,5.38025181819553));
#17017=CARTESIAN_POINT('Ctrl Pts',(2.78,2.6,5.36678788880707));
#17018=CARTESIAN_POINT('',(2.7,2.52,5.36678788880707));
#17019=CARTESIAN_POINT('',(2.69829980684391,2.52001806864527,5.40717967697245));
#17020=CARTESIAN_POINT('Ctrl Pts',(2.7,2.52,5.36678788880707));
#17021=CARTESIAN_POINT('Ctrl Pts',(2.7,2.52,5.38025181819553));
#17022=CARTESIAN_POINT('Ctrl Pts',(2.69942945076934,2.51999405556084,5.39371574758399));
#17023=CARTESIAN_POINT('Ctrl Pts',(2.69829980684391,2.52001806864527,5.40717967697245));
#17024=CARTESIAN_POINT('',(2.78,2.6,5.40717967697245));
#17025=CARTESIAN_POINT('Origin',(-1.4375,2.58232233047034,8.66267766952966));
#17026=CARTESIAN_POINT('',(5.68306019374819,2.57387961250363,8.68306019374819));
#17027=CARTESIAN_POINT('',(4.88692077572932,2.01092403125258,10.0421551930181));
#17028=CARTESIAN_POINT('',(3.29248197949184,3.56408953076227,6.29248197949182));
#17029=CARTESIAN_POINT('',(-3.45077738091134,3.49852142863302,6.45077738091131));
#17030=CARTESIAN_POINT('Origin',(5.66267766952966,2.58232233047034,5.46875));
#17031=CARTESIAN_POINT('',(6.3287007863016,2.3064465226494,8.30485269104902));
#17032=CARTESIAN_POINT('Origin',(5.75,2.52,8.67));
#17033=CARTESIAN_POINT('Origin',(-0.675,2.58232233047034,0.0873223304703362));
#17034=CARTESIAN_POINT('',(-3.77888057658085,3.36261663512876,1.97111942341917));
#17035=CARTESIAN_POINT('',(-3.36446283715638,2.82138175573458,0.664462837156383));
#17036=CARTESIAN_POINT('Origin',(-5.66267766952966,2.58232233047034,3.28125));
#17037=CARTESIAN_POINT('',(-5.70535533905933,2.56464466094067,3.28125));
#17038=CARTESIAN_POINT('Origin',(-2.78732233047034,2.58232233047034,4.70625));
#17039=CARTESIAN_POINT('',(-2.83,2.6,5.36678788880707));
#17040=CARTESIAN_POINT('Ctrl Pts',(-2.74464466094067,2.56464466094067,5.36678788880707));
#17041=CARTESIAN_POINT('Ctrl Pts',(-2.74464466094067,2.56464466094067,5.37716630475529));
#17042=CARTESIAN_POINT('Ctrl Pts',(-2.74456950540286,2.56471935013259,5.38754472070352));
#17043=CARTESIAN_POINT('Ctrl Pts',(-2.74442178368681,2.56486895213672,5.39792313665175));
#17044=CARTESIAN_POINT('Ctrl Pts',(-2.77309644062712,2.57642977396045,5.36678788880707));
#17045=CARTESIAN_POINT('Ctrl Pts',(-2.77309644062712,2.57642977396045,5.37716630475529));
#17046=CARTESIAN_POINT('Ctrl Pts',(-2.77304633693524,2.57647956675506,5.38754472070352));
#17047=CARTESIAN_POINT('Ctrl Pts',(-2.77294785579121,2.57657930142448,5.39792313665175));
#17048=CARTESIAN_POINT('Ctrl Pts',(-2.80154822031356,2.58821488698022,5.36678788880707));
#17049=CARTESIAN_POINT('Ctrl Pts',(-2.80154822031356,2.58821488698022,5.37716630475529));
#17050=CARTESIAN_POINT('Ctrl Pts',(-2.80152316846762,2.58823978337753,5.38754472070352));
#17051=CARTESIAN_POINT('Ctrl Pts',(-2.8014739278956,2.58828965071224,5.39792313665175));
#17052=CARTESIAN_POINT('Ctrl Pts',(-2.83,2.6,5.36678788880707));
#17053=CARTESIAN_POINT('Ctrl Pts',(-2.83,2.6,5.37716630475529));
#17054=CARTESIAN_POINT('Ctrl Pts',(-2.83,2.6,5.38754472070352));
#17055=CARTESIAN_POINT('Ctrl Pts',(-2.83,2.6,5.39792313665175));
#17056=CARTESIAN_POINT('',(-2.74442178368681,2.56486895213672,5.39792313665175));
#17057=CARTESIAN_POINT('Ctrl Pts',(-2.83,2.6,5.39792313665175));
#17058=CARTESIAN_POINT('Ctrl Pts',(-2.8014739278956,2.58828965071224,5.39792313665175));
#17059=CARTESIAN_POINT('Ctrl Pts',(-2.77294785579121,2.57657930142448,5.39792313665175));
#17060=CARTESIAN_POINT('Ctrl Pts',(-2.74442178368681,2.56486895213672,5.39792313665175));
#17061=CARTESIAN_POINT('Ctrl Pts',(-2.74442178368681,2.56486895213672,5.39792313665175));
#17062=CARTESIAN_POINT('Ctrl Pts',(-2.74456950540286,2.56471935013259,5.38754472070352));
#17063=CARTESIAN_POINT('Ctrl Pts',(-2.74464466094067,2.56464466094067,5.37716630475529));
#17064=CARTESIAN_POINT('Ctrl Pts',(-2.74464466094067,2.56464466094067,5.36678788880707));
#17065=CARTESIAN_POINT('Ctrl Pts',(-2.83,2.6,5.39792313665175));
#17066=CARTESIAN_POINT('Ctrl Pts',(-2.81333333333333,2.6,5.40100865009198));
#17067=CARTESIAN_POINT('Ctrl Pts',(-2.79666666666667,2.6,5.40409416353221));
#17068=CARTESIAN_POINT('Ctrl Pts',(-2.78,2.6,5.40717967697245));
#17069=CARTESIAN_POINT('Ctrl Pts',(-2.8014739278956,2.58828965071224,5.39792313665175));
#17070=CARTESIAN_POINT('Ctrl Pts',(-2.7942866733878,2.59219347080718,5.40100865009198));
#17071=CARTESIAN_POINT('Ctrl Pts',(-2.78712438474266,2.59609711969564,5.40409416353221));
#17072=CARTESIAN_POINT('Ctrl Pts',(-2.78,2.6,5.40717967697245));
#17073=CARTESIAN_POINT('Ctrl Pts',(-2.77294785579121,2.57657930142448,5.39792313665175));
#17074=CARTESIAN_POINT('Ctrl Pts',(-2.77524001344226,2.58438694161436,5.40100865009198));
#17075=CARTESIAN_POINT('Ctrl Pts',(-2.77758210281866,2.59219423939128,5.40409416353221));
#17076=CARTESIAN_POINT('Ctrl Pts',(-2.78,2.6,5.40717967697245));
#17077=CARTESIAN_POINT('Ctrl Pts',(-2.74442178368681,2.56486895213672,5.39792313665175));
#17078=CARTESIAN_POINT('Ctrl Pts',(-2.75619335349672,2.57658041242155,5.40100865009198));
#17079=CARTESIAN_POINT('Ctrl Pts',(-2.76803982089465,2.58829135908692,5.40409416353221));
#17080=CARTESIAN_POINT('Ctrl Pts',(-2.78,2.6,5.40717967697245));
#17081=CARTESIAN_POINT('Ctrl Pts',(-2.78,2.6,5.40717967697245));
#17082=CARTESIAN_POINT('Ctrl Pts',(-2.76803982089465,2.58829135908692,5.40409416353221));
#17083=CARTESIAN_POINT('Ctrl Pts',(-2.75619335349672,2.57658041242155,5.40100865009198));
#17084=CARTESIAN_POINT('Ctrl Pts',(-2.74442178368681,2.56486895213672,5.39792313665175));
#17085=CARTESIAN_POINT('Origin',(-4.6,2.57,7.75));
#17086=CARTESIAN_POINT('',(-4.93,2.54,7.75));
#17087=CARTESIAN_POINT('',(-4.96,2.57,7.75));
#17088=CARTESIAN_POINT('Origin',(-4.6,2.54,7.75));
#17089=CARTESIAN_POINT('Origin',(-4.6,0.,7.75));
#17090=CARTESIAN_POINT('',(-4.93,-2.54,7.75));
#17091=CARTESIAN_POINT('Origin',(-4.6,-2.54,7.75));
#17092=CARTESIAN_POINT('',(-4.93,0.,7.75));
#17093=CARTESIAN_POINT('Origin',(-4.6,-2.57,7.75));
#17094=CARTESIAN_POINT('',(-4.96,-2.57,7.75));
#17095=CARTESIAN_POINT('Origin',(4.6,2.57,1.));
#17096=CARTESIAN_POINT('',(4.27,2.54,1.));
#17097=CARTESIAN_POINT('',(4.24,2.57,1.));
#17098=CARTESIAN_POINT('Origin',(4.6,2.54,1.));
#17099=CARTESIAN_POINT('Origin',(4.6,0.,1.));
#17100=CARTESIAN_POINT('',(4.27,-2.54,1.));
#17101=CARTESIAN_POINT('Origin',(4.6,-2.54,1.));
#17102=CARTESIAN_POINT('',(4.27,0.,1.));
#17103=CARTESIAN_POINT('Origin',(4.6,-2.57,1.));
#17104=CARTESIAN_POINT('',(4.24,-2.57,1.));
#17105=CARTESIAN_POINT('Origin',(4.6,2.57,7.75));
#17106=CARTESIAN_POINT('',(4.27,2.54,7.75));
#17107=CARTESIAN_POINT('',(4.24,2.57,7.75));
#17108=CARTESIAN_POINT('Origin',(4.6,2.54,7.75));
#17109=CARTESIAN_POINT('Origin',(4.6,0.,7.75));
#17110=CARTESIAN_POINT('',(4.27,-2.54,7.75));
#17111=CARTESIAN_POINT('Origin',(4.6,-2.54,7.75));
#17112=CARTESIAN_POINT('',(4.27,0.,7.75));
#17113=CARTESIAN_POINT('Origin',(4.6,-2.57,7.75));
#17114=CARTESIAN_POINT('',(4.24,-2.57,7.75));
#17115=CARTESIAN_POINT('Origin',(-4.6,2.57,1.));
#17116=CARTESIAN_POINT('',(-4.93,2.54,1.));
#17117=CARTESIAN_POINT('',(-4.96,2.57,1.));
#17118=CARTESIAN_POINT('Origin',(-4.6,2.54,1.));
#17119=CARTESIAN_POINT('Origin',(-4.6,0.,1.));
#17120=CARTESIAN_POINT('',(-4.93,-2.54,1.));
#17121=CARTESIAN_POINT('Origin',(-4.6,-2.54,1.));
#17122=CARTESIAN_POINT('',(-4.93,0.,1.));
#17123=CARTESIAN_POINT('Origin',(-4.6,-2.57,1.));
#17124=CARTESIAN_POINT('',(-4.96,-2.57,1.));
#17125=CARTESIAN_POINT('Origin',(0.,0.,5.7));
#17126=CARTESIAN_POINT('',(-1.35,-1.65327317884893E-16,5.7));
#17127=CARTESIAN_POINT('Origin',(0.,0.,5.7));
#17128=CARTESIAN_POINT('',(-1.3,-1.59204083889156E-16,5.75));
#17129=CARTESIAN_POINT('',(-1.35,-1.65327317884893E-16,5.7));
#17130=CARTESIAN_POINT('Origin',(0.,0.,5.75));
#17131=CARTESIAN_POINT('Origin',(0.,0.,6.125));
#17132=CARTESIAN_POINT('',(-1.3,-1.59204083889156E-16,6.5));
#17133=CARTESIAN_POINT('',(-1.3,-1.59204083889156E-16,6.125));
#17134=CARTESIAN_POINT('Origin',(0.,0.,6.5));
#17135=CARTESIAN_POINT('Origin',(0.7,0.,6.5));
#17136=CARTESIAN_POINT('',(-0.7,-8.57252759403147E-17,6.5));
#17137=CARTESIAN_POINT('Origin',(0.,0.,6.5));
#17138=CARTESIAN_POINT('Origin',(0.,0.,7.225));
#17139=CARTESIAN_POINT('',(-0.7,-8.57252759403147E-17,7.95));
#17140=CARTESIAN_POINT('',(-0.7,-8.57252759403147E-17,7.225));
#17141=CARTESIAN_POINT('Origin',(0.,0.,7.95));
#17142=CARTESIAN_POINT('Origin',(1.3,0.,7.95));
#17143=CARTESIAN_POINT('',(-1.3,-1.59204083889156E-16,7.95));
#17144=CARTESIAN_POINT('Origin',(0.,0.,7.95));
#17145=CARTESIAN_POINT('Origin',(0.,0.,8.325));
#17146=CARTESIAN_POINT('',(-1.3,-1.59204083889156E-16,8.7));
#17147=CARTESIAN_POINT('',(-1.3,-1.59204083889156E-16,8.325));
#17148=CARTESIAN_POINT('Origin',(0.,0.,8.7));
#17149=CARTESIAN_POINT('Origin',(0.,0.,8.75));
#17150=CARTESIAN_POINT('',(-1.35,1.65327317884893E-16,8.75));
#17151=CARTESIAN_POINT('',(-1.35,-1.65327317884893E-16,8.75));
#17152=CARTESIAN_POINT('Origin',(0.,0.,8.75));
#17153=CARTESIAN_POINT('Origin',(-2.7,0.,3.));
#17154=CARTESIAN_POINT('',(-2.75,-1.59204083889156E-16,1.7));
#17155=CARTESIAN_POINT('',(-2.7,-1.65327317884893E-16,1.65));
#17156=CARTESIAN_POINT('Origin',(-2.75,0.,3.));
#17157=CARTESIAN_POINT('Origin',(-3.125,0.,3.));
#17158=CARTESIAN_POINT('',(-3.5,-1.59204083889156E-16,1.7));
#17159=CARTESIAN_POINT('',(-3.125,-1.59204083889156E-16,1.7));
#17160=CARTESIAN_POINT('Origin',(-3.5,0.,3.));
#17161=CARTESIAN_POINT('Origin',(-3.5,0.,3.7));
#17162=CARTESIAN_POINT('',(-3.5,-8.57252759403147E-17,2.3));
#17163=CARTESIAN_POINT('Origin',(-3.5,0.,3.));
#17164=CARTESIAN_POINT('Origin',(-4.225,0.,3.));
#17165=CARTESIAN_POINT('',(-4.95,-8.57252759403147E-17,2.3));
#17166=CARTESIAN_POINT('',(-4.225,-8.57252759403147E-17,2.3));
#17167=CARTESIAN_POINT('Origin',(-4.95,0.,3.));
#17168=CARTESIAN_POINT('Origin',(-4.95,0.,4.3));
#17169=CARTESIAN_POINT('',(-4.95,-1.59204083889156E-16,1.7));
#17170=CARTESIAN_POINT('Origin',(-4.95,0.,3.));
#17171=CARTESIAN_POINT('Origin',(-5.325,0.,3.));
#17172=CARTESIAN_POINT('',(-5.7,-1.59204083889156E-16,1.7));
#17173=CARTESIAN_POINT('',(-5.325,-1.59204083889156E-16,1.7));
#17174=CARTESIAN_POINT('Origin',(-5.7,0.,3.));
#17175=CARTESIAN_POINT('Origin',(-5.75,0.,3.));
#17176=CARTESIAN_POINT('',(-5.75,-1.65327317884893E-16,1.65));
#17177=CARTESIAN_POINT('Origin',(5.75,0.,3.));
#17178=CARTESIAN_POINT('',(5.7,-1.59204083889156E-16,1.7));
#17179=CARTESIAN_POINT('',(5.75,-1.65327317884893E-16,1.65));
#17180=CARTESIAN_POINT('Origin',(5.7,0.,3.));
#17181=CARTESIAN_POINT('Origin',(5.325,0.,3.));
#17182=CARTESIAN_POINT('',(4.95,-1.59204083889156E-16,1.7));
#17183=CARTESIAN_POINT('',(5.325,-1.59204083889156E-16,1.7));
#17184=CARTESIAN_POINT('Origin',(4.95,0.,3.));
#17185=CARTESIAN_POINT('Origin',(4.95,0.,3.7));
#17186=CARTESIAN_POINT('',(4.95,-8.57252759403147E-17,2.3));
#17187=CARTESIAN_POINT('Origin',(4.95,0.,3.));
#17188=CARTESIAN_POINT('Origin',(4.225,0.,3.));
#17189=CARTESIAN_POINT('',(3.5,-8.57252759403147E-17,2.3));
#17190=CARTESIAN_POINT('',(4.225,-8.57252759403147E-17,2.3));
#17191=CARTESIAN_POINT('Origin',(3.5,0.,3.));
#17192=CARTESIAN_POINT('Origin',(3.5,0.,4.3));
#17193=CARTESIAN_POINT('',(3.5,-1.59204083889156E-16,1.7));
#17194=CARTESIAN_POINT('Origin',(3.5,0.,3.));
#17195=CARTESIAN_POINT('Origin',(3.125,0.,3.));
#17196=CARTESIAN_POINT('',(2.75,-1.59204083889156E-16,1.7));
#17197=CARTESIAN_POINT('',(3.125,-1.59204083889156E-16,1.7));
#17198=CARTESIAN_POINT('Origin',(2.75,0.,3.));
#17199=CARTESIAN_POINT('Origin',(2.7,0.,3.));
#17200=CARTESIAN_POINT('',(2.7,-1.65327317884893E-16,1.65));
#17201=CARTESIAN_POINT('Ctrl Pts',(-2.31142159057266,-2.58116161377225,
5.9781544825592));
#17202=CARTESIAN_POINT('Ctrl Pts',(-2.36128434130633,-2.56784999958484,
5.93183474087413));
#17203=CARTESIAN_POINT('Ctrl Pts',(-2.43995511674461,-2.5495376072066,5.86291013494394));
#17204=CARTESIAN_POINT('Ctrl Pts',(-2.53391137386914,-2.53448278521197,
5.76471507012624));
#17205=CARTESIAN_POINT('Ctrl Pts',(-2.59241291603181,-2.52736920010306,
5.69068137785945));
#17206=CARTESIAN_POINT('Ctrl Pts',(-2.64432087785964,-2.52278488329719,
5.60511511887677));
#17207=CARTESIAN_POINT('Ctrl Pts',(-2.68329779044149,-2.52048776381013,
5.50684199397487));
#17208=CARTESIAN_POINT('Ctrl Pts',(-2.69557514809684,-2.5200759873036,5.43965416929022));
#17209=CARTESIAN_POINT('Ctrl Pts',(-2.69829980684391,-2.52001806864527,
5.40717967697245));
#17210=CARTESIAN_POINT('Ctrl Pts',(-2.34899533776733,-2.58744107584817,
6.01494078908382));
#17211=CARTESIAN_POINT('Ctrl Pts',(-2.39865683979399,-2.5785666663899,5.96728981679977));
#17212=CARTESIAN_POINT('Ctrl Pts',(-2.4766857923441,-2.5663584048044,5.89405976020693));
#17213=CARTESIAN_POINT('Ctrl Pts',(-2.56915127374486,-2.55632185680798,
5.78808953647345));
#17214=CARTESIAN_POINT('Ctrl Pts',(-2.62632274601193,-2.55157946673537,
5.70829633719456));
#17215=CARTESIAN_POINT('Ctrl Pts',(-2.67648636529298,-2.54852325553146,
5.61659793937325));
#17216=CARTESIAN_POINT('Ctrl Pts',(-2.71319808109984,-2.54699184254009,
5.51215507085786));
#17217=CARTESIAN_POINT('Ctrl Pts',(-2.72371676539789,-2.54671732486907,
5.44131770509747));
#17218=CARTESIAN_POINT('Ctrl Pts',(-2.7255332045626,-2.54667871243018,5.40717967697245));
#17219=CARTESIAN_POINT('Ctrl Pts',(-2.38656908496201,-2.59372053792408,
6.05172709560844));
#17220=CARTESIAN_POINT('Ctrl Pts',(-2.43602933828165,-2.58928333319495,
6.0027448927254));
#17221=CARTESIAN_POINT('Ctrl Pts',(-2.5134164679436,-2.5831792024022,5.92520938546991));
#17222=CARTESIAN_POINT('Ctrl Pts',(-2.60439117362058,-2.57816092840399,
5.81146400282065));
#17223=CARTESIAN_POINT('Ctrl Pts',(-2.66023257599205,-2.57578973336769,
5.72591129652966));
#17224=CARTESIAN_POINT('Ctrl Pts',(-2.70865185272632,-2.57426162776573,
5.62808075986973));
#17225=CARTESIAN_POINT('Ctrl Pts',(-2.7430983717582,-2.57349592127004,5.51746814774084));
#17226=CARTESIAN_POINT('Ctrl Pts',(-2.75185838269895,-2.57335866243453,
5.44298124090471));
#17227=CARTESIAN_POINT('Ctrl Pts',(-2.7527666022813,-2.57333935621509,5.40717967697245));
#17228=CARTESIAN_POINT('Ctrl Pts',(-2.42414283215669,-2.6,6.08851340213307));
#17229=CARTESIAN_POINT('Ctrl Pts',(-2.47340183676932,-2.6,6.03819996865104));
#17230=CARTESIAN_POINT('Ctrl Pts',(-2.55014714354309,-2.6,5.9563590107329));
#17231=CARTESIAN_POINT('Ctrl Pts',(-2.6396310734963,-2.6,5.83483846916786));
#17232=CARTESIAN_POINT('Ctrl Pts',(-2.69414240597218,-2.6,5.74352625586477));
#17233=CARTESIAN_POINT('Ctrl Pts',(-2.74081734015966,-2.6,5.6395635803662));
#17234=CARTESIAN_POINT('Ctrl Pts',(-2.77299866241655,-2.6,5.52278122462383));
#17235=CARTESIAN_POINT('Ctrl Pts',(-2.78,-2.6,5.44464477671195));
#17236=CARTESIAN_POINT('Ctrl Pts',(-2.78,-2.6,5.40717967697245));
#17237=CARTESIAN_POINT('',(-2.31142159057266,-2.58116161377225,5.9781544825592));
#17238=CARTESIAN_POINT('Ctrl Pts',(-2.31142159057266,-2.58116161377225,
5.9781544825592));
#17239=CARTESIAN_POINT('Ctrl Pts',(-2.34899533776733,-2.58744107584817,
6.01494078908382));
#17240=CARTESIAN_POINT('Ctrl Pts',(-2.38656908496201,-2.59372053792408,
6.05172709560844));
#17241=CARTESIAN_POINT('Ctrl Pts',(-2.42414283215669,-2.6,6.08851340213307));
#17242=CARTESIAN_POINT('Ctrl Pts',(-2.69829980684391,-2.52001806864527,
5.40717967697245));
#17243=CARTESIAN_POINT('Ctrl Pts',(-2.69557514809684,-2.5200759873036,5.43965416929022));
#17244=CARTESIAN_POINT('Ctrl Pts',(-2.68329779044149,-2.52048776381013,
5.50684199397487));
#17245=CARTESIAN_POINT('Ctrl Pts',(-2.64432087785964,-2.52278488329719,
5.60511511887677));
#17246=CARTESIAN_POINT('Ctrl Pts',(-2.59241291603181,-2.52736920010306,
5.69068137785945));
#17247=CARTESIAN_POINT('Ctrl Pts',(-2.53391137386914,-2.53448278521197,
5.76471507012624));
#17248=CARTESIAN_POINT('Ctrl Pts',(-2.43995511674461,-2.5495376072066,5.86291013494394));
#17249=CARTESIAN_POINT('Ctrl Pts',(-2.36128434130633,-2.56784999958484,
5.93183474087413));
#17250=CARTESIAN_POINT('Ctrl Pts',(-2.31142159057266,-2.58116161377225,
5.9781544825592));
#17251=CARTESIAN_POINT('Ctrl Pts',(2.31142159057333,2.58116161377208,5.97815448255858));
#17252=CARTESIAN_POINT('Ctrl Pts',(2.36128434130696,2.56784999958469,5.93183474087357));
#17253=CARTESIAN_POINT('Ctrl Pts',(2.46729918759723,2.54332863292027,5.83885512810807));
#17254=CARTESIAN_POINT('Ctrl Pts',(2.56567273666995,2.53021793080961,5.72941144954258));
#17255=CARTESIAN_POINT('Ctrl Pts',(2.63596652889653,2.52334815894777,5.62089094351626));
#17256=CARTESIAN_POINT('Ctrl Pts',(2.68071920404472,2.52052866674434,5.52338620228086));
#17257=CARTESIAN_POINT('Ctrl Pts',(2.69557514809684,2.5200759873036,5.43965416929018));
#17258=CARTESIAN_POINT('Ctrl Pts',(2.69829980684391,2.52001806864527,5.40717967697245));
#17259=CARTESIAN_POINT('Ctrl Pts',(2.348995337768,2.58744107584805,6.01494078908319));
#17260=CARTESIAN_POINT('Ctrl Pts',(2.39865683979462,2.57856666638979,5.96728981679918));
#17261=CARTESIAN_POINT('Ctrl Pts',(2.50379036101454,2.56221908861351,5.86841726345666));
#17262=CARTESIAN_POINT('Ctrl Pts',(2.60032540397316,2.55347862053974,5.74988540376893));
#17263=CARTESIAN_POINT('Ctrl Pts',(2.66846922987872,2.54889877263185,5.63346263613916));
#17264=CARTESIAN_POINT('Ctrl Pts',(2.7110544394694,2.54701911116289,5.52956123521929));
#17265=CARTESIAN_POINT('Ctrl Pts',(2.72371676539789,2.54671732486907,5.44131770509742));
#17266=CARTESIAN_POINT('Ctrl Pts',(2.7255332045626,2.54667871243018,5.40717967697245));
#17267=CARTESIAN_POINT('Ctrl Pts',(2.38656908496267,2.59372053792403,6.05172709560779));
#17268=CARTESIAN_POINT('Ctrl Pts',(2.43602933828227,2.5892833331949,6.00274489272478));
#17269=CARTESIAN_POINT('Ctrl Pts',(2.54028153443185,2.58110954430676,5.89797939880525));
#17270=CARTESIAN_POINT('Ctrl Pts',(2.63497807127636,2.57673931026987,5.77035935799528));
#17271=CARTESIAN_POINT('Ctrl Pts',(2.70097193086091,2.57444938631592,5.64603432876207));
#17272=CARTESIAN_POINT('Ctrl Pts',(2.74138967489408,2.57350955558144,5.53573626815772));
#17273=CARTESIAN_POINT('Ctrl Pts',(2.75185838269895,2.57335866243453,5.44298124090466));
#17274=CARTESIAN_POINT('Ctrl Pts',(2.7527666022813,2.57333935621509,5.40717967697245));
#17275=CARTESIAN_POINT('Ctrl Pts',(2.42414283215735,2.6,6.0885134021324));
#17276=CARTESIAN_POINT('Ctrl Pts',(2.47340183676993,2.6,6.03819996865039));
#17277=CARTESIAN_POINT('Ctrl Pts',(2.57677270784915,2.6,5.92754153415384));
#17278=CARTESIAN_POINT('Ctrl Pts',(2.66963073857957,2.6,5.79083331222164));
#17279=CARTESIAN_POINT('Ctrl Pts',(2.7334746318431,2.6,5.65860602138498));
#17280=CARTESIAN_POINT('Ctrl Pts',(2.77172491031876,2.6,5.54191130109615));
#17281=CARTESIAN_POINT('Ctrl Pts',(2.78,2.6,5.44464477671191));
#17282=CARTESIAN_POINT('Ctrl Pts',(2.78,2.6,5.40717967697245));
#17283=CARTESIAN_POINT('',(2.31142159057333,2.58116161377208,5.97815448255858));
#17284=CARTESIAN_POINT('Ctrl Pts',(2.31142159057333,2.58116161377208,5.97815448255858));
#17285=CARTESIAN_POINT('Ctrl Pts',(2.348995337768,2.58744107584805,6.01494078908319));
#17286=CARTESIAN_POINT('Ctrl Pts',(2.38656908496267,2.59372053792403,6.05172709560779));
#17287=CARTESIAN_POINT('Ctrl Pts',(2.42414283215735,2.6,6.0885134021324));
#17288=CARTESIAN_POINT('Ctrl Pts',(2.69829980684391,2.52001806864527,5.40717967697245));
#17289=CARTESIAN_POINT('Ctrl Pts',(2.69557514809684,2.5200759873036,5.43965416929018));
#17290=CARTESIAN_POINT('Ctrl Pts',(2.68071920404472,2.52052866674434,5.52338620228086));
#17291=CARTESIAN_POINT('Ctrl Pts',(2.63596652889653,2.52334815894777,5.62089094351626));
#17292=CARTESIAN_POINT('Ctrl Pts',(2.56567273666995,2.53021793080961,5.72941144954258));
#17293=CARTESIAN_POINT('Ctrl Pts',(2.46729918759723,2.54332863292027,5.83885512810807));
#17294=CARTESIAN_POINT('Ctrl Pts',(2.36128434130696,2.56784999958469,5.93183474087357));
#17295=CARTESIAN_POINT('Ctrl Pts',(2.31142159057333,2.58116161377208,5.97815448255858));
#17296=CARTESIAN_POINT('Origin',(-2.74,0.,0.04));
#17297=CARTESIAN_POINT('Origin',(-5.71,0.,0.04));
#17298=CARTESIAN_POINT('Origin',(5.71,0.,0.04));
#17299=CARTESIAN_POINT('Origin',(2.74,0.,0.04));
#17300=CARTESIAN_POINT('Origin',(2.74,2.56,2.1875));
#17301=CARTESIAN_POINT('Origin',(-5.71,2.56,2.1875));
#17302=CARTESIAN_POINT('Origin',(-2.74,-2.56,5.0375));
#17303=CARTESIAN_POINT('Ctrl Pts',(2.69829980684391,-2.52001806864527,5.40717967697245));
#17304=CARTESIAN_POINT('Ctrl Pts',(2.69528352551617,-2.52008218638766,5.44312994227118));
#17305=CARTESIAN_POINT('Ctrl Pts',(2.68123989111592,-2.52051013648877,5.51729816380893));
#17306=CARTESIAN_POINT('Ctrl Pts',(2.63367794162332,-2.52356953989164,5.62595269195354));
#17307=CARTESIAN_POINT('Ctrl Pts',(2.55608221571234,-2.53094020120163,5.74414944732199));
#17308=CARTESIAN_POINT('Ctrl Pts',(2.47881891560007,-2.54263648495202,5.82345543387705));
#17309=CARTESIAN_POINT('Ctrl Pts',(2.38591323923068,-2.56211985755297,5.91035968403401));
#17310=CARTESIAN_POINT('Ctrl Pts',(2.34794220819964,-2.57141188347425,5.9442288456962));
#17311=CARTESIAN_POINT('Ctrl Pts',(2.31142159080892,-2.58116161370918,5.97815448233973));
#17312=CARTESIAN_POINT('Ctrl Pts',(2.7255332045626,-2.54667871243018,5.40717967697245));
#17313=CARTESIAN_POINT('Ctrl Pts',(2.72353019295656,-2.54670588833705,5.44500465970129));
#17314=CARTESIAN_POINT('Ctrl Pts',(2.71140788262801,-2.54701636077182,5.52317099586011));
#17315=CARTESIAN_POINT('Ctrl Pts',(2.66629357290831,-2.54905511343735,5.63884881308445));
#17316=CARTESIAN_POINT('Ctrl Pts',(2.59103946170864,-2.55395127036495,5.76578291819495));
#17317=CARTESIAN_POINT('Ctrl Pts',(2.51499306415409,-2.56181835630172,5.8516058289363));
#17318=CARTESIAN_POINT('Ctrl Pts',(2.4230785617572,-2.57470877665646,5.94444781460691));
#17319=CARTESIAN_POINT('Ctrl Pts',(2.38536381613614,-2.5809733210315,5.98001412068834));
#17320=CARTESIAN_POINT('Ctrl Pts',(2.34899533800264,-2.58744107580612,6.01494078885804));
#17321=CARTESIAN_POINT('Ctrl Pts',(2.7527666022813,-2.57333935621509,5.40717967697245));
#17322=CARTESIAN_POINT('Ctrl Pts',(2.75175333255962,-2.57337629805061,5.4467799812886));
#17323=CARTESIAN_POINT('Ctrl Pts',(2.7415821395726,-2.57349377571695,5.52908162910424));
#17324=CARTESIAN_POINT('Ctrl Pts',(2.6989137440639,-2.57451442645429,5.65177067977436));
#17325=CARTESIAN_POINT('Ctrl Pts',(2.62597409522993,-2.57698893083669,5.78730964038079));
#17326=CARTESIAN_POINT('Ctrl Pts',(2.55119649000168,-2.58081812865031,5.87997558417632));
#17327=CARTESIAN_POINT('Ctrl Pts',(2.4602196462861,-2.58741108089651,5.9783727139586));
#17328=CARTESIAN_POINT('Ctrl Pts',(2.42279964439558,-2.59043856244275,6.01587741917045));
#17329=CARTESIAN_POINT('Ctrl Pts',(2.38656908519636,-2.59372053790306,6.05172709537636));
#17330=CARTESIAN_POINT('Ctrl Pts',(2.78,-2.6,5.40717967697245));
#17331=CARTESIAN_POINT('Ctrl Pts',(2.78,-2.6,5.44865469871872));
#17332=CARTESIAN_POINT('Ctrl Pts',(2.77175013108469,-2.6,5.53495446115542));
#17333=CARTESIAN_POINT('Ctrl Pts',(2.73152937534889,-2.6,5.66466680090526));
#17334=CARTESIAN_POINT('Ctrl Pts',(2.66093134122623,-2.6,5.80894311125375));
#17335=CARTESIAN_POINT('Ctrl Pts',(2.5873706385557,-2.6,5.90812597923557));
#17336=CARTESIAN_POINT('Ctrl Pts',(2.49738496881261,-2.6,6.0124608445315));
#17337=CARTESIAN_POINT('Ctrl Pts',(2.46022125233207,-2.6,6.05166269416259));
#17338=CARTESIAN_POINT('Ctrl Pts',(2.42414283239008,-2.6,6.08851340189468));
#17339=CARTESIAN_POINT('',(2.31142159080892,-2.58116161370918,5.97815448233973));
#17340=CARTESIAN_POINT('Ctrl Pts',(2.42414283239008,-2.6,6.08851340189468));
#17341=CARTESIAN_POINT('Ctrl Pts',(2.38656908519636,-2.59372053790306,6.05172709537636));
#17342=CARTESIAN_POINT('Ctrl Pts',(2.34899533800264,-2.58744107580612,6.01494078885804));
#17343=CARTESIAN_POINT('Ctrl Pts',(2.31142159080892,-2.58116161370918,5.97815448233973));
#17344=CARTESIAN_POINT('',(2.69829980684391,-2.52001806864527,5.40717967697245));
#17345=CARTESIAN_POINT('Ctrl Pts',(2.31142159080892,-2.58116161370918,5.97815448233973));
#17346=CARTESIAN_POINT('Ctrl Pts',(2.34794220819964,-2.57141188347425,5.9442288456962));
#17347=CARTESIAN_POINT('Ctrl Pts',(2.38591323923068,-2.56211985755297,5.91035968403401));
#17348=CARTESIAN_POINT('Ctrl Pts',(2.47881891560007,-2.54263648495202,5.82345543387705));
#17349=CARTESIAN_POINT('Ctrl Pts',(2.55608221571234,-2.53094020120163,5.74414944732199));
#17350=CARTESIAN_POINT('Ctrl Pts',(2.63367794162332,-2.52356953989164,5.62595269195354));
#17351=CARTESIAN_POINT('Ctrl Pts',(2.68123989111592,-2.52051013648877,5.51729816380893));
#17352=CARTESIAN_POINT('Ctrl Pts',(2.69528352551617,-2.52008218638766,5.44312994227118));
#17353=CARTESIAN_POINT('Ctrl Pts',(2.69829980684391,-2.52001806864527,5.40717967697245));
#17354=CARTESIAN_POINT('',(2.69829980684391,-2.52001806864527,5.40717967697245));
#17355=CARTESIAN_POINT('Ctrl Pts',(2.7,-2.52,5.36678788880707));
#17356=CARTESIAN_POINT('Ctrl Pts',(2.7,-2.52,5.38025181819553));
#17357=CARTESIAN_POINT('Ctrl Pts',(2.69942945076934,-2.51999405556084,5.39371574758399));
#17358=CARTESIAN_POINT('Ctrl Pts',(2.69829980684391,-2.52001806864527,5.40717967697245));
#17359=CARTESIAN_POINT('Ctrl Pts',(2.72666666666667,-2.54666666666667,5.36678788880707));
#17360=CARTESIAN_POINT('Ctrl Pts',(2.72666666666667,-2.54666666666667,5.38025181819553));
#17361=CARTESIAN_POINT('Ctrl Pts',(2.72628630051289,-2.54666270370723,5.39371574758399));
#17362=CARTESIAN_POINT('Ctrl Pts',(2.7255332045626,-2.54667871243018,5.40717967697245));
#17363=CARTESIAN_POINT('Ctrl Pts',(2.75333333333333,-2.57333333333333,5.36678788880707));
#17364=CARTESIAN_POINT('Ctrl Pts',(2.75333333333333,-2.57333333333333,5.38025181819553));
#17365=CARTESIAN_POINT('Ctrl Pts',(2.75314315025645,-2.57333135185361,5.39371574758399));
#17366=CARTESIAN_POINT('Ctrl Pts',(2.7527666022813,-2.57333935621509,5.40717967697245));
#17367=CARTESIAN_POINT('Ctrl Pts',(2.78,-2.6,5.36678788880707));
#17368=CARTESIAN_POINT('Ctrl Pts',(2.78,-2.6,5.38025181819553));
#17369=CARTESIAN_POINT('Ctrl Pts',(2.78,-2.6,5.39371574758399));
#17370=CARTESIAN_POINT('Ctrl Pts',(2.78,-2.6,5.40717967697245));
#17371=CARTESIAN_POINT('Ctrl Pts',(2.69829980684391,-2.52001806864527,5.40717967697245));
#17372=CARTESIAN_POINT('Ctrl Pts',(2.69942945076934,-2.51999405556084,5.39371574758399));
#17373=CARTESIAN_POINT('Ctrl Pts',(2.7,-2.52,5.38025181819553));
#17374=CARTESIAN_POINT('Ctrl Pts',(2.7,-2.52,5.36678788880707));
#17375=CARTESIAN_POINT('Ctrl Pts',(-2.69829980684391,2.52001806864527,5.40717967697245));
#17376=CARTESIAN_POINT('Ctrl Pts',(-2.69528352551617,2.52008218638766,5.44312994227118));
#17377=CARTESIAN_POINT('Ctrl Pts',(-2.68123989111592,2.52051013648877,5.51729816380893));
#17378=CARTESIAN_POINT('Ctrl Pts',(-2.63367794162332,2.52356953989164,5.62595269195354));
#17379=CARTESIAN_POINT('Ctrl Pts',(-2.55608221571234,2.53094020120163,5.744149447322));
#17380=CARTESIAN_POINT('Ctrl Pts',(-2.47881891560007,2.54263648495202,5.82345543387705));
#17381=CARTESIAN_POINT('Ctrl Pts',(-2.38591323923047,2.56211985755302,5.91035968403422));
#17382=CARTESIAN_POINT('Ctrl Pts',(-2.34794220819919,2.57141188347436,5.9442288456966));
#17383=CARTESIAN_POINT('Ctrl Pts',(-2.31142159080827,2.58116161370936,5.97815448234033));
#17384=CARTESIAN_POINT('Ctrl Pts',(-2.7255332045626,2.54667871243018,5.40717967697245));
#17385=CARTESIAN_POINT('Ctrl Pts',(-2.72353019295656,2.54670588833705,5.44500465970129));
#17386=CARTESIAN_POINT('Ctrl Pts',(-2.71140788262801,2.54701636077182,5.52317099586011));
#17387=CARTESIAN_POINT('Ctrl Pts',(-2.66629357290831,2.54905511343735,5.63884881308445));
#17388=CARTESIAN_POINT('Ctrl Pts',(-2.59103946170864,2.55395127036495,5.76578291819496));
#17389=CARTESIAN_POINT('Ctrl Pts',(-2.51499306415409,2.56181835630172,5.8516058289363));
#17390=CARTESIAN_POINT('Ctrl Pts',(-2.42307856175698,2.5747087766565,5.94444781460713));
#17391=CARTESIAN_POINT('Ctrl Pts',(-2.38536381613569,2.58097332103158,5.98001412068877));
#17392=CARTESIAN_POINT('Ctrl Pts',(-2.34899533800199,2.58744107580624,6.01494078885867));
#17393=CARTESIAN_POINT('Ctrl Pts',(-2.7527666022813,2.57333935621509,5.40717967697245));
#17394=CARTESIAN_POINT('Ctrl Pts',(-2.75175333255962,2.57337629805061,5.4467799812886));
#17395=CARTESIAN_POINT('Ctrl Pts',(-2.74158213957261,2.57349377571695,5.52908162910424));
#17396=CARTESIAN_POINT('Ctrl Pts',(-2.69891374406391,2.57451442645429,5.65177067977436));
#17397=CARTESIAN_POINT('Ctrl Pts',(-2.62597409522993,2.57698893083669,5.78730964038079));
#17398=CARTESIAN_POINT('Ctrl Pts',(-2.55119649000168,2.58081812865031,5.87997558417632));
#17399=CARTESIAN_POINT('Ctrl Pts',(-2.46021964628589,2.58741108089653,5.97837271395883));
#17400=CARTESIAN_POINT('Ctrl Pts',(-2.42279964439514,2.59043856244278,6.01587741917089));
#17401=CARTESIAN_POINT('Ctrl Pts',(-2.38656908519572,2.59372053790312,6.051727095377));
#17402=CARTESIAN_POINT('Ctrl Pts',(-2.78,2.6,5.40717967697245));
#17403=CARTESIAN_POINT('Ctrl Pts',(-2.78,2.6,5.44865469871872));
#17404=CARTESIAN_POINT('Ctrl Pts',(-2.77175013108469,2.6,5.53495446115542));
#17405=CARTESIAN_POINT('Ctrl Pts',(-2.7315293753489,2.6,5.66466680090526));
#17406=CARTESIAN_POINT('Ctrl Pts',(-2.66093134122624,2.6,5.80894311125375));
#17407=CARTESIAN_POINT('Ctrl Pts',(-2.5873706385557,2.6,5.90812597923557));
#17408=CARTESIAN_POINT('Ctrl Pts',(-2.4973849688124,2.6,6.01246084453175));
#17409=CARTESIAN_POINT('Ctrl Pts',(-2.46022125233163,2.6,6.05166269416306));
#17410=CARTESIAN_POINT('Ctrl Pts',(-2.42414283238944,2.6,6.08851340189533));
#17411=CARTESIAN_POINT('',(-2.31142159080827,2.58116161370936,5.97815448234033));
#17412=CARTESIAN_POINT('Ctrl Pts',(-2.42414283238944,2.6,6.08851340189533));
#17413=CARTESIAN_POINT('Ctrl Pts',(-2.38656908519572,2.59372053790312,6.051727095377));
#17414=CARTESIAN_POINT('Ctrl Pts',(-2.34899533800199,2.58744107580624,6.01494078885867));
#17415=CARTESIAN_POINT('Ctrl Pts',(-2.31142159080827,2.58116161370936,5.97815448234033));
#17416=CARTESIAN_POINT('',(-2.69829980684391,2.52001806864527,5.40717967697245));
#17417=CARTESIAN_POINT('Ctrl Pts',(-2.31142159080827,2.58116161370936,5.97815448234033));
#17418=CARTESIAN_POINT('Ctrl Pts',(-2.34794220819919,2.57141188347436,5.9442288456966));
#17419=CARTESIAN_POINT('Ctrl Pts',(-2.38591323923047,2.56211985755302,5.91035968403422));
#17420=CARTESIAN_POINT('Ctrl Pts',(-2.47881891560007,2.54263648495202,5.82345543387705));
#17421=CARTESIAN_POINT('Ctrl Pts',(-2.55608221571234,2.53094020120163,5.744149447322));
#17422=CARTESIAN_POINT('Ctrl Pts',(-2.63367794162332,2.52356953989164,5.62595269195354));
#17423=CARTESIAN_POINT('Ctrl Pts',(-2.68123989111592,2.52051013648877,5.51729816380893));
#17424=CARTESIAN_POINT('Ctrl Pts',(-2.69528352551617,2.52008218638766,5.44312994227118));
#17425=CARTESIAN_POINT('Ctrl Pts',(-2.69829980684391,2.52001806864527,5.40717967697245));
#17426=CARTESIAN_POINT('',(-2.69829980684391,2.52001806864527,5.40717967697245));
#17427=CARTESIAN_POINT('Ctrl Pts',(-2.7,2.52,5.36678788880707));
#17428=CARTESIAN_POINT('Ctrl Pts',(-2.7,2.52,5.38025181819553));
#17429=CARTESIAN_POINT('Ctrl Pts',(-2.69942945076934,2.51999405556084,5.39371574758399));
#17430=CARTESIAN_POINT('Ctrl Pts',(-2.69829980684391,2.52001806864527,5.40717967697245));
#17431=CARTESIAN_POINT('Ctrl Pts',(-2.72666666666667,2.54666666666667,5.36678788880707));
#17432=CARTESIAN_POINT('Ctrl Pts',(-2.72666666666667,2.54666666666667,5.38025181819553));
#17433=CARTESIAN_POINT('Ctrl Pts',(-2.72628630051289,2.54666270370723,5.39371574758399));
#17434=CARTESIAN_POINT('Ctrl Pts',(-2.7255332045626,2.54667871243018,5.40717967697245));
#17435=CARTESIAN_POINT('Ctrl Pts',(-2.75333333333333,2.57333333333333,5.36678788880707));
#17436=CARTESIAN_POINT('Ctrl Pts',(-2.75333333333333,2.57333333333333,5.38025181819553));
#17437=CARTESIAN_POINT('Ctrl Pts',(-2.75314315025645,2.57333135185361,5.39371574758399));
#17438=CARTESIAN_POINT('Ctrl Pts',(-2.7527666022813,2.57333935621509,5.40717967697245));
#17439=CARTESIAN_POINT('Ctrl Pts',(-2.78,2.6,5.36678788880707));
#17440=CARTESIAN_POINT('Ctrl Pts',(-2.78,2.6,5.38025181819553));
#17441=CARTESIAN_POINT('Ctrl Pts',(-2.78,2.6,5.39371574758399));
#17442=CARTESIAN_POINT('Ctrl Pts',(-2.78,2.6,5.40717967697245));
#17443=CARTESIAN_POINT('Ctrl Pts',(-2.69829980684391,2.52001806864527,5.40717967697245));
#17444=CARTESIAN_POINT('Ctrl Pts',(-2.69942945076934,2.51999405556084,5.39371574758399));
#17445=CARTESIAN_POINT('Ctrl Pts',(-2.7,2.52,5.38025181819553));
#17446=CARTESIAN_POINT('Ctrl Pts',(-2.7,2.52,5.36678788880707));
#17447=CARTESIAN_POINT('Ctrl Pts',(-2.31142159057266,-2.58116161377225,
5.9781544825592));
#17448=CARTESIAN_POINT('Ctrl Pts',(-2.30761542875944,-2.59362449027802,
6.01749838383513));
#17449=CARTESIAN_POINT('Ctrl Pts',(-2.30380771440082,-2.6,6.05874632271281));
#17450=CARTESIAN_POINT('Ctrl Pts',(-2.3,-2.6,6.1));
#17451=CARTESIAN_POINT('Ctrl Pts',(-2.34899533776733,-2.58744107584817,
6.01494078908382));
#17452=CARTESIAN_POINT('Ctrl Pts',(-2.33266424854111,-2.59574966018535,
6.04244634525299));
#17453=CARTESIAN_POINT('Ctrl Pts',(-2.31633212428463,-2.6,6.07122125982333));
#17454=CARTESIAN_POINT('Ctrl Pts',(-2.3,-2.6,6.1));
#17455=CARTESIAN_POINT('Ctrl Pts',(-2.38656908496201,-2.59372053792408,
6.05172709560844));
#17456=CARTESIAN_POINT('Ctrl Pts',(-2.35771306832278,-2.59787483009267,
6.06739430667085));
#17457=CARTESIAN_POINT('Ctrl Pts',(-2.32885653416843,-2.6,6.08369619693384));
#17458=CARTESIAN_POINT('Ctrl Pts',(-2.3,-2.6,6.1));
#17459=CARTESIAN_POINT('Ctrl Pts',(-2.42414283215669,-2.6,6.08851340213307));
#17460=CARTESIAN_POINT('Ctrl Pts',(-2.38276188810446,-2.6,6.09234226808871));
#17461=CARTESIAN_POINT('Ctrl Pts',(-2.34138094405223,-2.6,6.09617113404436));
#17462=CARTESIAN_POINT('Ctrl Pts',(-2.3,-2.6,6.1));
#17463=CARTESIAN_POINT('Ctrl Pts',(-2.31142159057266,-2.58116161377225,
5.9781544825592));
#17464=CARTESIAN_POINT('Ctrl Pts',(-2.30761542875944,-2.59362449027802,
6.01749838383513));
#17465=CARTESIAN_POINT('Ctrl Pts',(-2.30380771440082,-2.6,6.05874632271281));
#17466=CARTESIAN_POINT('Ctrl Pts',(-2.3,-2.6,6.1));
#17467=CARTESIAN_POINT('Ctrl Pts',(2.31142159057333,2.58116161377208,5.97815448255858));
#17468=CARTESIAN_POINT('Ctrl Pts',(2.30761542875988,2.59362449027796,6.0174983838347));
#17469=CARTESIAN_POINT('Ctrl Pts',(2.30380771440105,2.6,6.0587463227126));
#17470=CARTESIAN_POINT('Ctrl Pts',(2.3,2.6,6.1));
#17471=CARTESIAN_POINT('Ctrl Pts',(2.348995337768,2.58744107584805,6.01494078908319));
#17472=CARTESIAN_POINT('Ctrl Pts',(2.33266424854156,2.59574966018531,6.04244634525256));
#17473=CARTESIAN_POINT('Ctrl Pts',(2.31633212428485,2.6,6.07122125982311));
#17474=CARTESIAN_POINT('Ctrl Pts',(2.3,2.6,6.1));
#17475=CARTESIAN_POINT('Ctrl Pts',(2.38656908496267,2.59372053792403,6.05172709560779));
#17476=CARTESIAN_POINT('Ctrl Pts',(2.35771306832323,2.59787483009265,6.06739430667041));
#17477=CARTESIAN_POINT('Ctrl Pts',(2.32885653416865,2.6,6.08369619693362));
#17478=CARTESIAN_POINT('Ctrl Pts',(2.3,2.6,6.1));
#17479=CARTESIAN_POINT('Ctrl Pts',(2.42414283215735,2.6,6.0885134021324));
#17480=CARTESIAN_POINT('Ctrl Pts',(2.3827618881049,2.6,6.09234226808826));
#17481=CARTESIAN_POINT('Ctrl Pts',(2.34138094405245,2.6,6.09617113404413));
#17482=CARTESIAN_POINT('Ctrl Pts',(2.3,2.6,6.1));
#17483=CARTESIAN_POINT('Ctrl Pts',(2.31142159057333,2.58116161377208,5.97815448255858));
#17484=CARTESIAN_POINT('Ctrl Pts',(2.30761542875988,2.59362449027796,6.0174983838347));
#17485=CARTESIAN_POINT('Ctrl Pts',(2.30380771440105,2.6,6.0587463227126));
#17486=CARTESIAN_POINT('Ctrl Pts',(2.3,2.6,6.1));
#17487=CARTESIAN_POINT('Ctrl Pts',(2.42414283239008,-2.6,6.08851340189468));
#17488=CARTESIAN_POINT('Ctrl Pts',(2.38276188826005,-2.6,6.09234226792978));
#17489=CARTESIAN_POINT('Ctrl Pts',(2.34138094413003,-2.6,6.09617113396489));
#17490=CARTESIAN_POINT('Ctrl Pts',(2.3,-2.6,6.1));
#17491=CARTESIAN_POINT('Ctrl Pts',(2.38656908519636,-2.59372053790306,6.05172709537636));
#17492=CARTESIAN_POINT('Ctrl Pts',(2.35771306847904,-2.59787483008549,6.06739430651421));
#17493=CARTESIAN_POINT('Ctrl Pts',(2.32885653424655,-2.6,6.08369619685551));
#17494=CARTESIAN_POINT('Ctrl Pts',(2.3,-2.6,6.1));
#17495=CARTESIAN_POINT('Ctrl Pts',(2.34899533800264,-2.58744107580612,6.01494078885804));
#17496=CARTESIAN_POINT('Ctrl Pts',(2.33266424869802,-2.59574966017099,6.04244634509863));
#17497=CARTESIAN_POINT('Ctrl Pts',(2.31633212436308,-2.6,6.07122125974614));
#17498=CARTESIAN_POINT('Ctrl Pts',(2.3,-2.6,6.1));
#17499=CARTESIAN_POINT('Ctrl Pts',(2.31142159080892,-2.58116161370918,5.97815448233973));
#17500=CARTESIAN_POINT('Ctrl Pts',(2.30761542891701,-2.59362449025648,6.01749838368306));
#17501=CARTESIAN_POINT('Ctrl Pts',(2.30380771447961,-2.6,6.05874632263676));
#17502=CARTESIAN_POINT('Ctrl Pts',(2.3,-2.6,6.1));
#17503=CARTESIAN_POINT('Ctrl Pts',(2.3,-2.6,6.1));
#17504=CARTESIAN_POINT('Ctrl Pts',(2.30380771447961,-2.6,6.05874632263676));
#17505=CARTESIAN_POINT('Ctrl Pts',(2.30761542891701,-2.59362449025648,6.01749838368306));
#17506=CARTESIAN_POINT('Ctrl Pts',(2.31142159080892,-2.58116161370918,5.97815448233973));
#17507=CARTESIAN_POINT('Ctrl Pts',(-2.42414283238944,2.6,6.08851340189533));
#17508=CARTESIAN_POINT('Ctrl Pts',(-2.38276188825963,2.6,6.09234226793022));
#17509=CARTESIAN_POINT('Ctrl Pts',(-2.34138094412981,2.6,6.09617113396511));
#17510=CARTESIAN_POINT('Ctrl Pts',(-2.3,2.6,6.1));
#17511=CARTESIAN_POINT('Ctrl Pts',(-2.38656908519572,2.59372053790312,6.051727095377));
#17512=CARTESIAN_POINT('Ctrl Pts',(-2.35771306847861,2.59787483008551,6.06739430651464));
#17513=CARTESIAN_POINT('Ctrl Pts',(-2.32885653424634,2.6,6.08369619685573));
#17514=CARTESIAN_POINT('Ctrl Pts',(-2.3,2.6,6.1));
#17515=CARTESIAN_POINT('Ctrl Pts',(-2.34899533800199,2.58744107580624,6.01494078885867));
#17516=CARTESIAN_POINT('Ctrl Pts',(-2.33266424869759,2.59574966017103,6.04244634509906));
#17517=CARTESIAN_POINT('Ctrl Pts',(-2.31633212436287,2.6,6.07122125974635));
#17518=CARTESIAN_POINT('Ctrl Pts',(-2.3,2.6,6.1));
#17519=CARTESIAN_POINT('Ctrl Pts',(-2.31142159080827,2.58116161370936,5.97815448234033));
#17520=CARTESIAN_POINT('Ctrl Pts',(-2.30761542891658,2.59362449025654,6.01749838368348));
#17521=CARTESIAN_POINT('Ctrl Pts',(-2.30380771447939,2.6,6.05874632263697));
#17522=CARTESIAN_POINT('Ctrl Pts',(-2.3,2.6,6.1));
#17523=CARTESIAN_POINT('Ctrl Pts',(-2.3,2.6,6.1));
#17524=CARTESIAN_POINT('Ctrl Pts',(-2.30380771447939,2.6,6.05874632263697));
#17525=CARTESIAN_POINT('Ctrl Pts',(-2.30761542891658,2.59362449025654,6.01749838368348));
#17526=CARTESIAN_POINT('Ctrl Pts',(-2.31142159080827,2.58116161370936,5.97815448234033));
#17527=CARTESIAN_POINT('Origin',(-2.3,-2.2,6.1));
#17528=CARTESIAN_POINT('',(-2.3,-2.2,5.7));
#17529=CARTESIAN_POINT('Origin',(-2.3,-2.2,5.3));
#17530=CARTESIAN_POINT('Origin',(-2.3,-2.2,6.1));
#17531=CARTESIAN_POINT('Origin',(-2.3,2.2,6.1));
#17532=CARTESIAN_POINT('',(-2.3,2.2,5.7));
#17533=CARTESIAN_POINT('Origin',(-2.3,2.2,6.1));
#17534=CARTESIAN_POINT('Origin',(-2.3,2.2,5.3));
#17535=CARTESIAN_POINT('Origin',(-5.75,0.,8.75));
#17536=CARTESIAN_POINT('Origin',(2.3,2.2,6.1));
#17537=CARTESIAN_POINT('',(2.3,2.2,5.7));
#17538=CARTESIAN_POINT('Origin',(2.3,2.2,5.3));
#17539=CARTESIAN_POINT('Origin',(2.3,2.2,6.1));
#17540=CARTESIAN_POINT('Origin',(2.3,0.,5.3));
#17541=CARTESIAN_POINT('',(2.3,-2.2,5.7));
#17542=CARTESIAN_POINT('Origin',(2.3,-2.2,5.3));
#17543=CARTESIAN_POINT('',(2.3,0.,5.7));
#17544=CARTESIAN_POINT('Origin',(2.3,-2.2,6.1));
#17545=CARTESIAN_POINT('Origin',(2.3,-2.2,6.1));
#17546=CARTESIAN_POINT('Origin',(-2.3,0.,5.3));
#17547=CARTESIAN_POINT('',(-2.3,0.,5.7));
#17548=CARTESIAN_POINT('Origin',(1.35,2.2,6.1));
#17549=CARTESIAN_POINT('',(1.35,2.2,5.7));
#17550=CARTESIAN_POINT('Origin',(2.7,0.,5.7));
#17551=CARTESIAN_POINT('',(1.35,-2.2,5.7));
#17552=CARTESIAN_POINT('Origin',(1.35,-2.2,6.1));
#31614=UNCERTAINTY_MEASURE_WITH_UNIT(LENGTH_MEASURE(0.001),#31639,
'DISTANCE_ACCURACY_VALUE',
'Maximum model space distance between geometric entities at asserted c
onnectivities');
#31625=UNCERTAINTY_MEASURE_WITH_UNIT(LENGTH_MEASURE(0.001),#31639,
'DISTANCE_ACCURACY_VALUE',
'Maximum model space distance between geometric entities at asserted c
onnectivities');
#31627=(
GEOMETRIC_REPRESENTATION_CONTEXT(3)
GLOBAL_UNCERTAINTY_ASSIGNED_CONTEXT((#31614))
GLOBAL_UNIT_ASSIGNED_CONTEXT((#31639,#31641,#31642))
REPRESENTATION_CONTEXT('','3D')
);
#31638=(
GEOMETRIC_REPRESENTATION_CONTEXT(3)
GLOBAL_UNCERTAINTY_ASSIGNED_CONTEXT((#31625))
GLOBAL_UNIT_ASSIGNED_CONTEXT((#31639,#31641,#31642))
REPRESENTATION_CONTEXT('','3D')
);
#31639=(
LENGTH_UNIT()
NAMED_UNIT(*)
SI_UNIT(.CENTI.,.METRE.)
);
#31641=(
NAMED_UNIT(*)
PLANE_ANGLE_UNIT()
SI_UNIT($,.RADIAN.)
);
#31642=(
NAMED_UNIT(*)
SI_UNIT($,.STERADIAN.)
SOLID_ANGLE_UNIT()
);
#31644=SHAPE_DEFINITION_REPRESENTATION(#31656,#31705);
#31656=PRODUCT_DEFINITION_SHAPE('',$,#31718);
#31705=SHAPE_REPRESENTATION('',(#12614),#31627);
#31716=PRODUCT_DEFINITION_CONTEXT('part definition',#31754,'design');
#31718=PRODUCT_DEFINITION('2026-10-22-02-42-10-486',
'01_Aluminium_Gearbox_Frame_115x87.5x52',#31730,#31716);
#31730=PRODUCT_DEFINITION_FORMATION('',$,#31757);
#31754=APPLICATION_CONTEXT(
'Core Data for Automotive Mechanical Design Process');
#31755=PRODUCT_CONTEXT('part definition',#31754,'mechanical');
#31757=PRODUCT('2026-10-22-02-42-10-486',
'01_Aluminium_Gearbox_Frame_115x87.5x52',$,(#31755));
#31803=COLOUR_RGB('Dark Blue',0.08,0.2,0.34);
#31804=FILL_AREA_STYLE_COLOUR('',#31803);
#31805=FILL_AREA_STYLE('',(#31804));
#31806=SURFACE_STYLE_FILL_AREA(#31805);
#31807=SURFACE_SIDE_STYLE('',(#31806));
#31808=SURFACE_STYLE_USAGE(.BOTH.,#31807);
#31809=PRESENTATION_STYLE_ASSIGNMENT((#31808));
ENDSEC;
END-ISO-10303-21;
